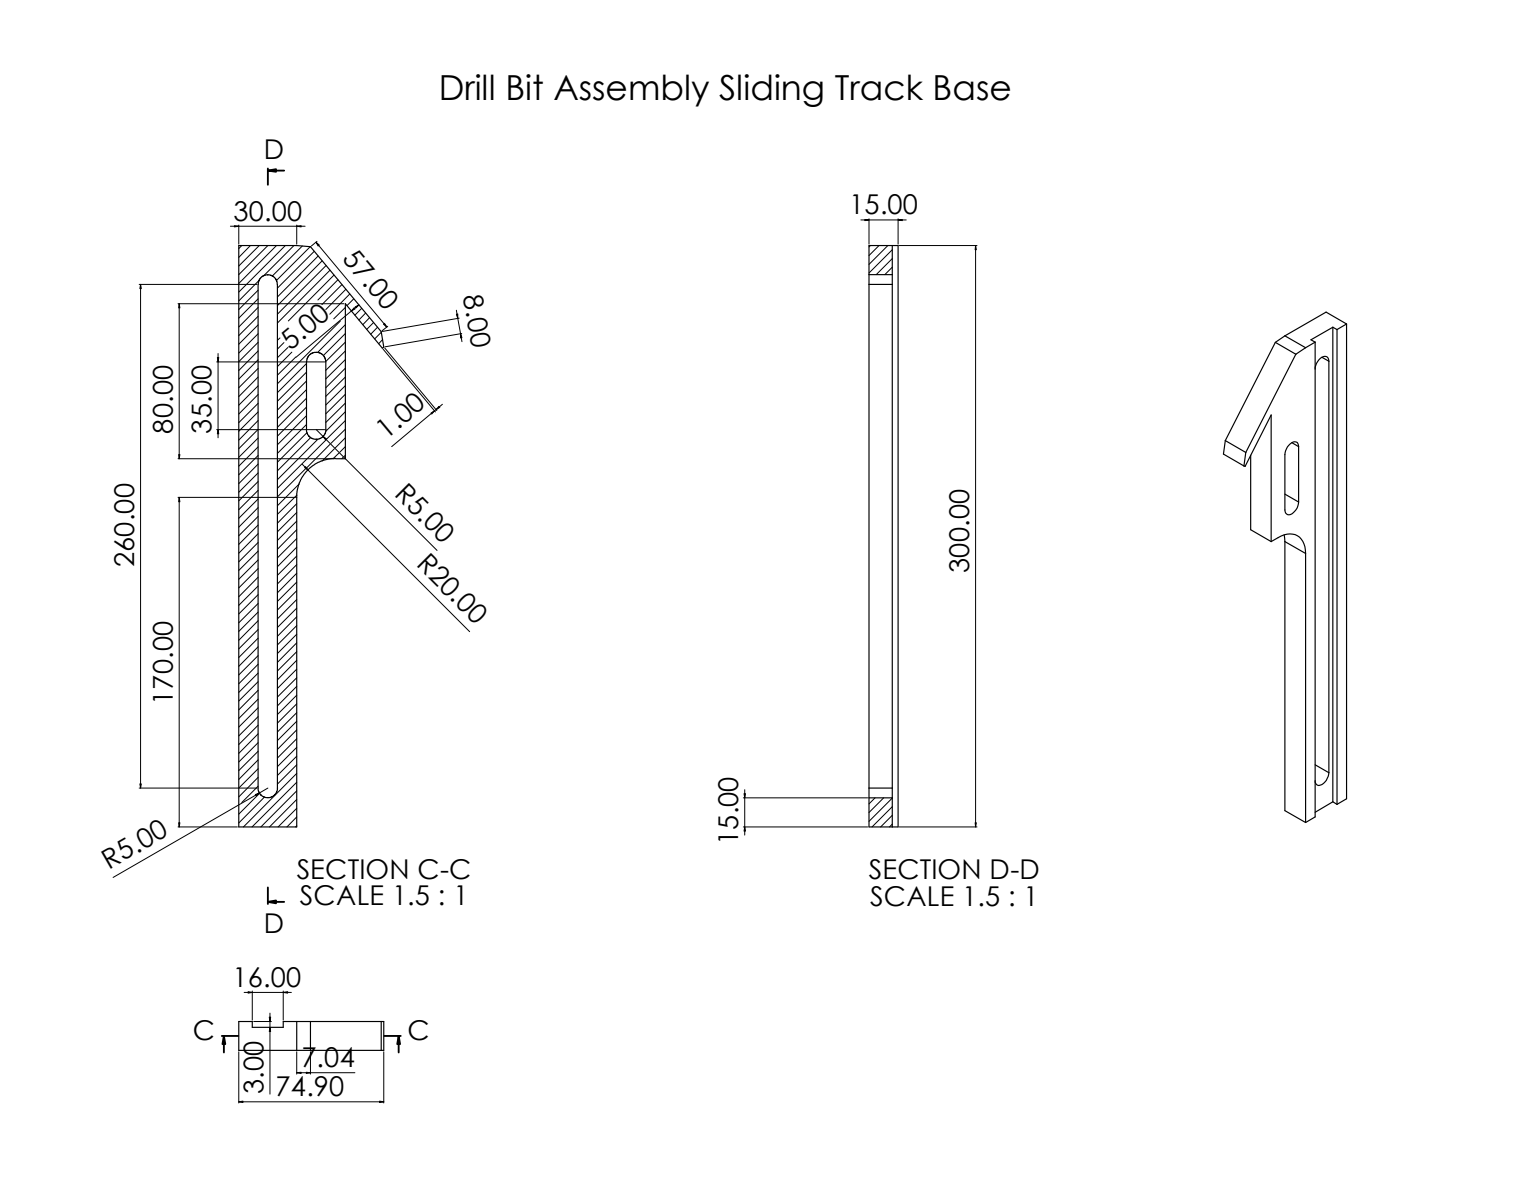
ISO-10303-21;
HEADER;
FILE_DESCRIPTION (('STEP AP214'),
    '1' );
FILE_NAME ('Drill Bit Assembly Sliding Track Base.step',
    '2026-10-26T22:46:44',
    ( '' ),
    ( '' ),
    'SwSTEP 2.0',
    'SolidWorks 2025',
    '' );
FILE_SCHEMA (( 'AUTOMOTIVE_DESIGN' ));
ENDSEC;

DATA;
#10=ORIENTED_EDGE ( 'NONE', *, *, #14818, .T. ) ;
#22=VECTOR ( 'NONE', #7023, 1000.000000000000114 ) ;
#42=CYLINDRICAL_SURFACE ( 'NONE', #6692, 5.000000000000002665 ) ;
#84=AXIS2_PLACEMENT_3D ( 'NONE', #10451, #8972, #10240 ) ;
#92=ORIENTED_EDGE ( 'NONE', *, *, #17549, .F. ) ;
#102=ADVANCED_FACE ( 'NONE', ( #18525 ), #10234, .F. ) ;
#113=ORIENTED_EDGE ( 'NONE', *, *, #4613, .F. ) ;
#117=DIRECTION ( 'NONE',  ( -0.5000000000000029976, 0.8660254037844370423, 0.000000000000000000 ) ) ;
#122=VERTEX_POINT ( 'NONE', #2105 ) ;
#123=APPLICATION_CONTEXT ( 'automotive_design' ) ;
#189=DIRECTION ( 'NONE',  ( -0.8660254037844360431, -0.5000000000000044409, 5.976026924694052093E-17 ) ) ;
#198=PLANE ( 'NONE',  #5711 ) ;
#204=DIRECTION ( 'NONE',  ( 0.8660254037844361541, 0.5000000000000043299, -5.976026924694053325E-17 ) ) ;
#209=ORIENTED_EDGE ( 'NONE', *, *, #20399, .T. ) ;
#222=FACE_OUTER_BOUND ( 'NONE', #14547, .T. ) ;
#243=UNCERTAINTY_MEASURE_WITH_UNIT (LENGTH_MEASURE( 1.000000000000000082E-05 ), #16702, 'distance_accuracy_value', 'NONE');
#300=LINE ( 'NONE', #11651, #4810 ) ;
#312=ORIENTED_EDGE ( 'NONE', *, *, #4694, .F. ) ;
#350=ORIENTED_EDGE ( 'NONE', *, *, #10318, .F. ) ;
#352=CARTESIAN_POINT ( 'NONE',  ( 69.50490953756755630, 173.5703347563769796, 16.00000000000001066 ) ) ;
#362=VECTOR ( 'NONE', #204, 1000.000000000000114 ) ;
#443=ADVANCED_FACE ( 'NONE', ( #4623 ), #13103, .F. ) ;
#466=FACE_OUTER_BOUND ( 'NONE', #2081, .T. ) ;
#469=CARTESIAN_POINT ( 'NONE',  ( 89.99529059433416478, 168.0799536996104848, 21.00000000000000711 ) ) ;
#494=ORIENTED_EDGE ( 'NONE', *, *, #20248, .T. ) ;
#495=FACE_OUTER_BOUND ( 'NONE', #6270, .T. ) ;
#509=ORIENTED_EDGE ( 'NONE', *, *, #2019, .T. ) ;
#517=FACE_OUTER_BOUND ( 'NONE', #17017, .T. ) ;
#524=ORIENTED_EDGE ( 'NONE', *, *, #10776, .F. ) ;
#540=CARTESIAN_POINT ( 'NONE',  ( 52.00490953756739287, 203.8812238888322383, 16.00000000000001066 ) ) ;
#544=DIRECTION ( 'NONE',  ( -1.153604387573317816E-16, 8.028960261725416899E-17, -1.000000000000000000 ) ) ;
#572=LINE ( 'NONE', #11705, #22 ) ;
#596=LINE ( 'NONE', #6053, #2836 ) ;
#604=LINE ( 'NONE', #7163, #17252 ) ;
#614=EDGE_LOOP ( 'NONE', ( #1540, #2040, #6697, #17636 ) ) ;
#640=DIRECTION ( 'NONE',  ( -0.8660254037844361541, -0.5000000000000043299, 0.000000000000000000 ) ) ;
#669=LINE ( 'NONE', #15217, #9538 ) ;
#715=VECTOR ( 'NONE', #14881, 1000.000000000000227 ) ;
#721=DIRECTION ( 'NONE',  ( 0.5000000000000044409, -0.8660254037844360431, -8.673617379884021914E-17 ) ) ;
#734=VERTEX_POINT ( 'NONE', #3213 ) ;
#740=CYLINDRICAL_SURFACE ( 'NONE', #13407, 5.000000000000005329 ) ;
#813=LINE ( 'NONE', #2095, #20345 ) ;
#814=EDGE_CURVE ( 'NONE', #5086, #6648, #7657, .T. ) ;
#817=CARTESIAN_POINT ( 'NONE',  ( 162.0049095375683237, 13.35563505625637859, -19.00000000000000355 ) ) ;
#843=EDGE_CURVE ( 'NONE', #19778, #2748, #14999, .T. ) ;
#873=EDGE_CURVE ( 'NONE', #9960, #7294, #7008, .T. ) ;
#877=AXIS2_PLACEMENT_3D ( 'NONE', #18226, #14549, #1913 ) ;
#909=CARTESIAN_POINT ( 'NONE',  ( 69.50490953756755630, 173.5703347563769796, 6.000000000000010658 ) ) ;
#943=CARTESIAN_POINT ( 'NONE',  ( 57.20986367771971004, 224.8659788670223634, 44.53282986889897899 ) ) ;
#953=ORIENTED_EDGE ( 'NONE', *, *, #3595, .F. ) ;
#988=DIRECTION ( 'NONE',  ( 0.3200921998322429629, -0.5544159532159284032, -0.7682212795973754060 ) ) ;
#1012=ADVANCED_FACE ( 'NONE', ( #2576 ), #12330, .F. ) ;
#1089=( NAMED_UNIT ( * ) PLANE_ANGLE_UNIT ( ) SI_UNIT ( $, .RADIAN. ) );
#1131=LINE ( 'NONE', #10862, #20660 ) ;
#1148=EDGE_CURVE ( 'NONE', #3117, #9960, #12846, .T. ) ;
#1195=DIRECTION ( 'NONE',  ( 0.8660254037844361541, 0.5000000000000043299, -5.976026924694053325E-17 ) ) ;
#1208=VERTEX_POINT ( 'NONE', #4575 ) ;
#1213=DIRECTION ( 'NONE',  ( -0.3841106397986904786, 0.6652991438591134843, -0.6401843996644803747 ) ) ;
#1218=VECTOR ( 'NONE', #4888, 999.9999999999998863 ) ;
#1274=DIRECTION ( 'NONE',  ( 0.000000000000000000, 0.000000000000000000, 1.000000000000000000 ) ) ;
#1325=PRODUCT_DEFINITION_FORMATION_WITH_SPECIFIED_SOURCE ( 'ANY', '', #20237, .NOT_KNOWN. ) ;
#1451=DIRECTION ( 'NONE',  ( -0.5000000000000043299, 0.8660254037844361541, 1.272130549049658454E-16 ) ) ;
#1474=EDGE_CURVE ( 'NONE', #10313, #10227, #2340, .T. ) ;
#1496=ADVANCED_FACE ( 'NONE', ( #13106 ), #11502, .F. ) ;
#1497=DIRECTION ( 'NONE',  ( -0.5000000000000029976, 0.8660254037844370423, 0.000000000000000000 ) ) ;
#1519=CARTESIAN_POINT ( 'NONE',  ( 182.3972143829816446, 2.035126980567696364, -22.00000000000003908 ) ) ;
#1520=CARTESIAN_POINT ( 'NONE',  ( 44.99529059433372424, 246.0222400402097946, -8.999999999999973355 ) ) ;
#1527=ORIENTED_EDGE ( 'NONE', *, *, #14882, .F. ) ;
#1540=ORIENTED_EDGE ( 'NONE', *, *, #15388, .T. ) ;
#1554=ORIENTED_EDGE ( 'NONE', *, *, #5736, .T. ) ;
#1582=EDGE_CURVE ( 'NONE', #4169, #5897, #12618, .T. ) ;
#1650=DIRECTION ( 'NONE',  ( -0.5000000000000029976, 0.8660254037844370423, 0.000000000000000000 ) ) ;
#1712=LINE ( 'NONE', #8374, #13909 ) ;
#1732=EDGE_CURVE ( 'NONE', #16063, #3717, #2384, .T. ) ;
#1744=VERTEX_POINT ( 'NONE', #5228 ) ;
#1750=VECTOR ( 'NONE', #9141, 1000.000000000000114 ) ;
#1757=CARTESIAN_POINT ( 'NONE',  ( 34.99529059433364608, 263.3427481158985302, -28.99999999999997513 ) ) ;
#1792=ORIENTED_EDGE ( 'NONE', *, *, #7559, .F. ) ;
#1808=CARTESIAN_POINT ( 'NONE',  ( 32.39721438298033007, 261.8427481158985302, -22.00000000000000355 ) ) ;
#1848=LINE ( 'NONE', #469, #12796 ) ;
#1871=DIRECTION ( 'NONE',  ( 0.000000000000000000, 0.000000000000000000, -1.000000000000000000 ) ) ;
#1882=VERTEX_POINT ( 'NONE', #18714 ) ;
#1912=AXIS2_PLACEMENT_3D ( 'NONE', #13249, #19798, #11757 ) ;
#1913=DIRECTION ( 'NONE',  ( 0.000000000000000000, -0.8108848540793835991, 0.5852057359806522863 ) ) ;
#1938=EDGE_LOOP ( 'NONE', ( #14408, #7446, #12643, #9895 ) ) ;
#1960=CARTESIAN_POINT ( 'NONE',  ( 57.20986367771984504, 224.8659788670219939, 44.53282986889903583 ) ) ;
#2019=EDGE_CURVE ( 'NONE', #19831, #13880, #17857, .T. ) ;
#2028=ORIENTED_EDGE ( 'NONE', *, *, #7150, .F. ) ;
#2040=ORIENTED_EDGE ( 'NONE', *, *, #1474, .T. ) ;
#2043=ORIENTED_EDGE ( 'NONE', *, *, #1582, .T. ) ;
#2081=EDGE_LOOP ( 'NONE', ( #19123, #6063, #19574, #13979 ) ) ;
#2095=CARTESIAN_POINT ( 'NONE',  ( 184.9952905943349606, 3.535126980567727450, -29.00000000000001066 ) ) ;
#2105=CARTESIAN_POINT ( 'NONE',  ( 48.16104799571871098, 210.5389873765740560, 45.89527237623691747 ) ) ;
#2141=CARTESIAN_POINT ( 'NONE',  ( 32.39721438298033007, 261.8427481158985302, -22.00000000000000355 ) ) ;
#2149=ORIENTED_EDGE ( 'NONE', *, *, #10776, .T. ) ;
#2205=CARTESIAN_POINT ( 'NONE',  ( 99.99529059433426426, 150.7594456239217777, 1.000000000000008438 ) ) ;
#2217=ORIENTED_EDGE ( 'NONE', *, *, #7593, .T. ) ;
#2260=EDGE_CURVE ( 'NONE', #15541, #9504, #13815, .T. ) ;
#2292=EDGE_CURVE ( 'NONE', #9960, #734, #10615, .T. ) ;
#2301=FACE_OUTER_BOUND ( 'NONE', #14390, .T. ) ;
#2312=ORIENTED_EDGE ( 'NONE', *, *, #2928, .T. ) ;
#2340=LINE ( 'NONE', #9202, #6212 ) ;
#2358=ORIENTED_EDGE ( 'NONE', *, *, #1732, .F. ) ;
#2380=DIRECTION ( 'NONE',  ( -0.8660254037844360431, -0.5000000000000044409, 5.976026924694052093E-17 ) ) ;
#2384=LINE ( 'NONE', #15235, #4553 ) ;
#2386=ADVANCED_FACE ( 'NONE', ( #18579 ), #12960, .F. ) ;
#2414=EDGE_CURVE ( 'NONE', #16240, #8157, #16622, .T. ) ;
#2430=CARTESIAN_POINT ( 'NONE',  ( 172.3972143829816162, 19.35563505625646030, -19.00000000000000355 ) ) ;
#2432=ORIENTED_EDGE ( 'NONE', *, *, #4613, .T. ) ;
#2442=VECTOR ( 'NONE', #7671, 1000.000000000000227 ) ;
#2489=ORIENTED_EDGE ( 'NONE', *, *, #3198, .T. ) ;
#2527=PLANE ( 'NONE',  #84 ) ;
#2547=ORIENTED_EDGE ( 'NONE', *, *, #20248, .F. ) ;
#2558=EDGE_CURVE ( 'NONE', #10285, #1208, #19571, .T. ) ;
#2576=FACE_OUTER_BOUND ( 'NONE', #5270, .T. ) ;
#2610=CARTESIAN_POINT ( 'NONE',  ( 87.00490953756771262, 143.2594456239216925, 1.000000000000009326 ) ) ;
#2620=ORIENTED_EDGE ( 'NONE', *, *, #11484, .T. ) ;
#2622=ORIENTED_EDGE ( 'NONE', *, *, #11749, .T. ) ;
#2631=ORIENTED_EDGE ( 'NONE', *, *, #15255, .T. ) ;
#2670=EDGE_LOOP ( 'NONE', ( #8116, #14442, #7233, #8193 ) ) ;
#2748=VERTEX_POINT ( 'NONE', #11956 ) ;
#2768=ORIENTED_EDGE ( 'NONE', *, *, #7687, .T. ) ;
#2775=VECTOR ( 'NONE', #1213, 1000.000000000000114 ) ;
#2780=VECTOR ( 'NONE', #15502, 1000.000000000000227 ) ;
#2836=VECTOR ( 'NONE', #7046, 1000.000000000000227 ) ;
#2837=EDGE_CURVE ( 'NONE', #3359, #10810, #9269, .T. ) ;
#2838=ORIENTED_EDGE ( 'NONE', *, *, #2843, .F. ) ;
#2843=EDGE_CURVE ( 'NONE', #3717, #5485, #15465, .T. ) ;
#2851=APPLICATION_CONTEXT ( 'automotive_design' ) ;
#2854=ORIENTED_EDGE ( 'NONE', *, *, #843, .T. ) ;
#2906=CARTESIAN_POINT ( 'NONE',  ( 22.32500173739930460, 255.2883321626825932, 8.042028396309257587 ) ) ;
#2918=EDGE_LOOP ( 'NONE', ( #509, #20075, #113, #10552 ) ) ;
#2928=EDGE_CURVE ( 'NONE', #2748, #10227, #18337, .T. ) ;
#2955=AXIS2_PLACEMENT_3D ( 'NONE', #19299, #7847, #1497 ) ;
#3005=LINE ( 'NONE', #1519, #7771 ) ;
#3034=LINE ( 'NONE', #15679, #13135 ) ;
#3039=DIRECTION ( 'NONE',  ( 0.5000000000000044409, -0.8660254037844360431, 0.000000000000000000 ) ) ;
#3102=VECTOR ( 'NONE', #7583, 999.9999999999998863 ) ;
#3113=FACE_OUTER_BOUND ( 'NONE', #19423, .T. ) ;
#3117=VERTEX_POINT ( 'NONE', #18277 ) ;
#3186=EDGE_CURVE ( 'NONE', #17982, #10285, #13517, .T. ) ;
#3196=DIRECTION ( 'NONE',  ( -0.8660254037844361541, -0.5000000000000045519, 5.976026924694053325E-17 ) ) ;
#3198=EDGE_CURVE ( 'NONE', #3359, #9504, #10629, .T. ) ;
#3205=CARTESIAN_POINT ( 'NONE',  ( 184.9952905943349606, 3.535126980567709687, -22.00000000000003908 ) ) ;
#3213=CARTESIAN_POINT ( 'NONE',  ( 22.00490953756710510, 255.8427481158984733, -28.99999999999997513 ) ) ;
#3218=ORIENTED_EDGE ( 'NONE', *, *, #843, .F. ) ;
#3232=DIRECTION ( 'NONE',  ( 0.8660254037844360431, 0.5000000000000044409, -5.976026924694053325E-17 ) ) ;
#3270=EDGE_CURVE ( 'NONE', #11034, #20099, #12561, .T. ) ;
#3286=CARTESIAN_POINT ( 'NONE',  ( 52.00490953756739287, 203.8812238888322383, 6.000000000000010658 ) ) ;
#3359=VERTEX_POINT ( 'NONE', #2906 ) ;
#3365=ORIENTED_EDGE ( 'NONE', *, *, #13197, .F. ) ;
#3370=CARTESIAN_POINT ( 'NONE',  ( 44.99529059433372424, 246.0222400402097946, -18.99999999999997513 ) ) ;
#3381=FACE_OUTER_BOUND ( 'NONE', #5314, .T. ) ;
#3390=CARTESIAN_POINT ( 'NONE',  ( 182.3972143829816446, 2.035126980567696364, -6.000000000000009770 ) ) ;
#3405=AXIS2_PLACEMENT_3D ( 'NONE', #14558, #17827, #15934 ) ;
#3412=ORIENTED_EDGE ( 'NONE', *, *, #17197, .F. ) ;
#3415=ORIENTED_EDGE ( 'NONE', *, *, #11618, .F. ) ;
#3417=VECTOR ( 'NONE', #14485, 1000.000000000000227 ) ;
#3440=CARTESIAN_POINT ( 'NONE',  ( 32.00490953756718682, 238.5222400402097094, -13.99999999999997335 ) ) ;
#3441=VECTOR ( 'NONE', #8435, 1000.000000000000114 ) ;
#3470=CARTESIAN_POINT ( 'NONE',  ( 32.00490953756718682, 238.5222400402097094, -18.99999999999997513 ) ) ;
#3473=DIRECTION ( 'NONE',  ( 0.5000000000000044409, -0.8660254037844360431, -8.673617379884021914E-17 ) ) ;
#3494=EDGE_CURVE ( 'NONE', #19831, #15541, #10642, .T. ) ;
#3511=ORIENTED_EDGE ( 'NONE', *, *, #17990, .T. ) ;
#3535=DIRECTION ( 'NONE',  ( 0.5000000000000046629, -0.8660254037844360431, 0.000000000000000000 ) ) ;
#3546=DIRECTION ( 'NONE',  ( -0.3200921998322431850, 0.5544159532159285142, 0.7682212795973754060 ) ) ;
#3559=AXIS2_PLACEMENT_3D ( 'NONE', #18463, #13907, #10606 ) ;
#3595=EDGE_CURVE ( 'NONE', #6648, #16240, #11289, .T. ) ;
#3609=CARTESIAN_POINT ( 'NONE',  ( 32.39721438298033007, 261.8427481158985302, -5.999999999999973355 ) ) ;
#3613=CARTESIAN_POINT ( 'NONE',  ( 46.88067919638974956, 212.7566511894377754, 48.96815749462641065 ) ) ;
#3644=( GEOMETRIC_REPRESENTATION_CONTEXT ( 3 ) GLOBAL_UNCERTAINTY_ASSIGNED_CONTEXT ( ( #16361 ) ) GLOBAL_UNIT_ASSIGNED_CONTEXT ( ( #12219, #1089, #15522 ) ) REPRESENTATION_CONTEXT ( 'NONE', 'WORKASPACE' ) );
#3645=( NAMED_UNIT ( * ) SI_UNIT ( $, .STERADIAN. ) SOLID_ANGLE_UNIT ( ) );
#3648=VECTOR ( 'NONE', #4240, 1000.000000000000227 ) ;
#3663=LINE ( 'NONE', #11635, #7812 ) ;
#3681=CARTESIAN_POINT ( 'NONE',  ( 32.39721438298033007, 261.8427481158985302, -5.999999999999973355 ) ) ;
#3705=VECTOR ( 'NONE', #20609, 1000.000000000000000 ) ;
#3717=VERTEX_POINT ( 'NONE', #18167 ) ;
#3723=DIRECTION ( 'NONE',  ( 0.5000000000000058842, -0.8660254037844352659, 0.000000000000000000 ) ) ;
#3735=ORIENTED_EDGE ( 'NONE', *, *, #4294, .F. ) ;
#3757=VERTEX_POINT ( 'NONE', #5535 ) ;
#3758=AXIS2_PLACEMENT_3D ( 'NONE', #9685, #6391, #3535 ) ;
#3776=DIRECTION ( 'NONE',  ( -0.000000000000000000, 4.625929269271485914E-16, -1.000000000000000000 ) ) ;
#3810=VERTEX_POINT ( 'NONE', #13932 ) ;
#3831=ORIENTED_EDGE ( 'NONE', *, *, #4082, .F. ) ;
#3868=CARTESIAN_POINT ( 'NONE',  ( -104.9618400369722622, 181.7992397999509819, 8.042028396309241600 ) ) ;
#3914=AXIS2_PLACEMENT_3D ( 'NONE', #15936, #4983, #4679 ) ;
#3939=AXIS2_PLACEMENT_3D ( 'NONE', #13181, #18468, #3723 ) ;
#4015=DIRECTION ( 'NONE',  ( 0.5000000000000041078, -0.8660254037844363761, 0.000000000000000000 ) ) ;
#4052=CARTESIAN_POINT ( 'NONE',  ( 82.49529059433407951, 181.0703347563770365, 16.00000000000001066 ) ) ;
#4065=CARTESIAN_POINT ( 'NONE',  ( 35.31538279416584913, 262.7883321626826501, 8.042028396309257587 ) ) ;
#4082=EDGE_CURVE ( 'NONE', #3117, #5485, #13375, .T. ) ;
#4118=ORIENTED_EDGE ( 'NONE', *, *, #3198, .F. ) ;
#4169=VERTEX_POINT ( 'NONE', #18359 ) ;
#4188=LINE ( 'NONE', #20716, #2442 ) ;
#4191=ORIENTED_EDGE ( 'NONE', *, *, #6008, .F. ) ;
#4205=CARTESIAN_POINT ( 'NONE',  ( 184.9952905943349606, 3.535126980567713240, 0.9999999999999876765 ) ) ;
#4220=LINE ( 'NONE', #5477, #17086 ) ;
#4239=CARTESIAN_POINT ( 'NONE',  ( 32.00490953756718682, 238.5222400402097094, -8.999999999999971578 ) ) ;
#4240=DIRECTION ( 'NONE',  ( -0.8660254037844360431, -0.5000000000000044409, 5.976026924694052093E-17 ) ) ;
#4294=EDGE_CURVE ( 'NONE', #3810, #16846, #9187, .T. ) ;
#4326=ORIENTED_EDGE ( 'NONE', *, *, #13282, .T. ) ;
#4364=CARTESIAN_POINT ( 'NONE',  ( 34.99529059433364608, 263.3427481158985302, -28.99999999999997513 ) ) ;
#4378=ORIENTED_EDGE ( 'NONE', *, *, #16152, .T. ) ;
#4400=CARTESIAN_POINT ( 'NONE',  ( 174.9952905943348469, 20.85563505625644609, -9.000000000000007105 ) ) ;
#4411=CARTESIAN_POINT ( 'NONE',  ( 20.40444853840588380, 258.6148278819781012, 4.841106397986906451 ) ) ;
#4439=DIRECTION ( 'NONE',  ( -5.175391130484829193E-17, -2.988013462347053780E-17, -1.000000000000000000 ) ) ;
#4475=ORIENTED_EDGE ( 'NONE', *, *, #4694, .T. ) ;
#4549=AXIS2_PLACEMENT_3D ( 'NONE', #12070, #20323, #10454 ) ;
#4553=VECTOR ( 'NONE', #16703, 1000.000000000000227 ) ;
#4575=CARTESIAN_POINT ( 'NONE',  ( 37.00490953756721524, 229.8619860023653985, 26.00000000000001776 ) ) ;
#4592=EDGE_CURVE ( 'NONE', #8802, #3117, #813, .T. ) ;
#4605=LINE ( 'NONE', #2610, #5814 ) ;
#4613=EDGE_CURVE ( 'NONE', #13544, #16413, #604, .T. ) ;
#4623=FACE_OUTER_BOUND ( 'NONE', #13097, .T. ) ;
#4629=FACE_OUTER_BOUND ( 'NONE', #14208, .T. ) ;
#4633=LINE ( 'NONE', #19160, #19626 ) ;
#4672=DIRECTION ( 'NONE',  ( -0.5000000000000043299, 0.8660254037844361541, 1.272130549049658700E-16 ) ) ;
#4679=DIRECTION ( 'NONE',  ( 0.5000000000000046629, -0.8660254037844360431, 0.000000000000000000 ) ) ;
#4693=ORIENTED_EDGE ( 'NONE', *, *, #10164, .T. ) ;
#4694=EDGE_CURVE ( 'NONE', #16413, #17073, #3005, .T. ) ;
#4720=DIRECTION ( 'NONE',  ( -0.5000000000000041078, 0.8660254037844363761, 0.000000000000000000 ) ) ;
#4770=AXIS2_PLACEMENT_3D ( 'NONE', #3868, #5657, #16709 ) ;
#4804=FACE_OUTER_BOUND ( 'NONE', #9235, .T. ) ;
#4810=VECTOR ( 'NONE', #18113, 1000.000000000000114 ) ;
#4818=ORIENTED_EDGE ( 'NONE', *, *, #16276, .F. ) ;
#4828=FACE_OUTER_BOUND ( 'NONE', #14732, .T. ) ;
#4862=DIRECTION ( 'NONE',  ( 0.5000000000000042188, -0.8660254037844361541, -1.067522139062650425E-16 ) ) ;
#4888=DIRECTION ( 'NONE',  ( 0.3841106397986906451, -0.6652991438591134843, 0.6401843996644803747 ) ) ;
#4948=DIRECTION ( 'NONE',  ( -0.5000000000000029976, 0.8660254037844370423, 0.000000000000000000 ) ) ;
#4983=DIRECTION ( 'NONE',  ( -0.8660254037844361541, -0.5000000000000045519, 5.976026924694053325E-17 ) ) ;
#5016=ORIENTED_EDGE ( 'NONE', *, *, #14063, .T. ) ;
#5082=CARTESIAN_POINT ( 'NONE',  ( 22.00490953756709800, 255.8427481158984733, 1.000000000000028644 ) ) ;
#5086=VERTEX_POINT ( 'NONE', #17294 ) ;
#5161=DIRECTION ( 'NONE',  ( 1.000000000000000000, 0.000000000000000000, -1.051300182579813185E-16 ) ) ;
#5198=ORIENTED_EDGE ( 'NONE', *, *, #9866, .T. ) ;
#5220=ORIENTED_EDGE ( 'NONE', *, *, #17144, .T. ) ;
#5221=DIRECTION ( 'NONE',  ( 0.8660254037844370423, 0.5000000000000027756, 1.765692291717890446E-15 ) ) ;
#5228=CARTESIAN_POINT ( 'NONE',  ( 77.00490953756764156, 160.5799536996104280, 26.00000000000001066 ) ) ;
#5229=ORIENTED_EDGE ( 'NONE', *, *, #1474, .F. ) ;
#5234=VERTEX_POINT ( 'NONE', #13676 ) ;
#5270=EDGE_LOOP ( 'NONE', ( #5198, #20606, #18436, #10211 ) ) ;
#5314=EDGE_LOOP ( 'NONE', ( #14238, #12408, #12374, #6867 ) ) ;
#5327=STYLED_ITEM('',(#20967),#17741);
#5428=CARTESIAN_POINT ( 'NONE',  ( 64.99529059433392320, 211.3812238888322952, 6.000000000000009770 ) ) ;
#5446=CARTESIAN_POINT ( 'NONE',  ( 61.15142905248526262, 218.0389873765740845, 45.89527237623694589 ) ) ;
#5454=DIRECTION ( 'NONE',  ( 0.5000000000000043299, -0.8660254037844361541, -1.214306433183764966E-16 ) ) ;
#5456=VECTOR ( 'NONE', #15711, 1000.000000000000000 ) ;
#5470=DIRECTION ( 'NONE',  ( -0.8660254037844361541, -0.5000000000000045519, 5.976026924694053325E-17 ) ) ;
#5477=CARTESIAN_POINT ( 'NONE',  ( 32.39721438298033007, 261.8427481158985302, -22.00000000000000355 ) ) ;
#5485=VERTEX_POINT ( 'NONE', #7817 ) ;
#5487=CARTESIAN_POINT ( 'NONE',  ( 34.99529059433364608, 263.3427481158985302, 1.000000000000028644 ) ) ;
#5503=ADVANCED_FACE ( 'NONE', ( #7612 ), #20539, .T. ) ;
#5535=CARTESIAN_POINT ( 'NONE',  ( 87.00490953756771262, 143.2594456239216925, 1.000000000000007772 ) ) ;
#5546=AXIS2_PLACEMENT_3D ( 'NONE', #17980, #3546, #10913 ) ;
#5551=EDGE_LOOP ( 'NONE', ( #2149, #11995, #3511, #13734, #2622 ) ) ;
#5580=PLANE ( 'NONE',  #4549 ) ;
#5611=VECTOR ( 'NONE', #11972, 1000.000000000000114 ) ;
#5613=EDGE_CURVE ( 'NONE', #10227, #20099, #17306, .T. ) ;
#5616=DIRECTION ( 'NONE',  ( -0.000000000000000000, 4.625929269271485914E-16, -1.000000000000000000 ) ) ;
#5657=DIRECTION ( 'NONE',  ( -0.4979466032338565329, 0.8624688162573705963, 0.09053574604251182767 ) ) ;
#5673=DIRECTION ( 'NONE',  ( -0.000000000000000000, 4.625929269271485914E-16, -1.000000000000000000 ) ) ;
#5678=CARTESIAN_POINT ( 'NONE',  ( 82.49529059433407951, 181.0703347563770365, 6.000000000000009770 ) ) ;
#5700=LINE ( 'NONE', #20448, #3648 ) ;
#5701=DIRECTION ( 'NONE',  ( -0.8660254037844360431, -0.5000000000000044409, 5.976026924694052093E-17 ) ) ;
#5704=CARTESIAN_POINT ( 'NONE',  ( 69.50490953756755630, 173.5703347563769796, 6.000000000000010658 ) ) ;
#5711=AXIS2_PLACEMENT_3D ( 'NONE', #11649, #6640, #14949 ) ;
#5736=EDGE_CURVE ( 'NONE', #13841, #3757, #16072, .T. ) ;
#5750=LINE ( 'NONE', #15550, #16856 ) ;
#5794=DIRECTION ( 'NONE',  ( -0.5000000000000041078, 0.8660254037844363761, 0.000000000000000000 ) ) ;
#5797=ORIENTED_EDGE ( 'NONE', *, *, #11749, .F. ) ;
#5814=VECTOR ( 'NONE', #7564, 1000.000000000000227 ) ;
#5883=CARTESIAN_POINT ( 'NONE',  ( 32.39721438298033007, 261.8427481158985302, -22.00000000000000355 ) ) ;
#5897=VERTEX_POINT ( 'NONE', #4052 ) ;
#5900=CARTESIAN_POINT ( 'NONE',  ( 44.99529059433372424, 246.0222400402097946, -8.999999999999973355 ) ) ;
#5901=ORIENTED_EDGE ( 'NONE', *, *, #11594, .F. ) ;
#5912=EDGE_CURVE ( 'NONE', #11034, #11090, #669, .T. ) ;
#5933=AXIS2_PLACEMENT_3D ( 'NONE', #11262, #3196, #6253 ) ;
#5957=VECTOR ( 'NONE', #17242, 1000.000000000000114 ) ;
#5959=CARTESIAN_POINT ( 'NONE',  ( 23.43933576707516053, 253.3582490066810919, 32.55737704917950737 ) ) ;
#5991=CARTESIAN_POINT ( 'NONE',  ( 57.20986367771982373, 224.8659788670219655, 44.53282986889902162 ) ) ;
#6008=EDGE_CURVE ( 'NONE', #14393, #17982, #7231, .T. ) ;
#6019=DIRECTION ( 'NONE',  ( 0.5000000000000045519, -0.8660254037844360431, -0.000000000000000000 ) ) ;
#6053=CARTESIAN_POINT ( 'NONE',  ( 82.49529059433407951, 181.0703347563770365, 16.00000000000001066 ) ) ;
#6060=DIRECTION ( 'NONE',  ( -1.218100516808353647E-16, 9.146065988991504310E-17, -1.000000000000000000 ) ) ;
#6063=ORIENTED_EDGE ( 'NONE', *, *, #8198, .F. ) ;
#6074=ORIENTED_EDGE ( 'NONE', *, *, #4294, .T. ) ;
#6161=VECTOR ( 'NONE', #1195, 1000.000000000000114 ) ;
#6212=VECTOR ( 'NONE', #5701, 1000.000000000000227 ) ;
#6253=DIRECTION ( 'NONE',  ( 0.5000000000000029976, -0.8660254037844370423, 0.000000000000000000 ) ) ;
#6270=EDGE_LOOP ( 'NONE', ( #8550, #16847, #4118, #350 ) ) ;
#6328=CARTESIAN_POINT ( 'NONE',  ( 32.00490953756718682, 238.5222400402097094, -8.999999999999971578 ) ) ;
#6341=ORIENTED_EDGE ( 'NONE', *, *, #7687, .F. ) ;
#6363=AXIS2_PLACEMENT_3D ( 'NONE', #1520, #6060, #12554 ) ;
#6370=ORIENTED_EDGE ( 'NONE', *, *, #18466, .F. ) ;
#6391=DIRECTION ( 'NONE',  ( -0.8660254037844360431, -0.5000000000000044409, 5.976026924694053325E-17 ) ) ;
#6439=CARTESIAN_POINT ( 'NONE',  ( 99.99529059433426426, 150.7594456239217777, 1.000000000000006883 ) ) ;
#6447=VECTOR ( 'NONE', #189, 1000.000000000000227 ) ;
#6481=CARTESIAN_POINT ( 'NONE',  ( 174.9952905943348469, 20.85563505625644609, -14.00000000000000533 ) ) ;
#6528=CARTESIAN_POINT ( 'NONE',  ( 37.00490953756721524, 229.8619860023653985, 26.00000000000001776 ) ) ;
#6539=VECTOR ( 'NONE', #4672, 1000.000000000000227 ) ;
#6554=VECTOR ( 'NONE', #6019, 1000.000000000000227 ) ;
#6572=CARTESIAN_POINT ( 'NONE',  ( 184.9952905943349606, 3.535126980567727450, -29.00000000000001066 ) ) ;
#6640=DIRECTION ( 'NONE',  ( -0.8660254037844361541, -0.5000000000000045519, 5.976026924694054558E-17 ) ) ;
#6648=VERTEX_POINT ( 'NONE', #18191 ) ;
#6665=LINE ( 'NONE', #16143, #15111 ) ;
#6692=AXIS2_PLACEMENT_3D ( 'NONE', #6481, #12982, #17855 ) ;
#6697=ORIENTED_EDGE ( 'NONE', *, *, #2928, .F. ) ;
#6731=ORIENTED_EDGE ( 'NONE', *, *, #7773, .T. ) ;
#6734=CARTESIAN_POINT ( 'NONE',  ( 69.50490953756755630, 173.5703347563769796, 11.00000000000001243 ) ) ;
#6745=CARTESIAN_POINT ( 'NONE',  ( 42.39721438298049350, 244.5222400402098231, -18.99999999999997513 ) ) ;
#6756=VECTOR ( 'NONE', #12549, 1000.000000000000000 ) ;
#6819=ADVANCED_FACE ( 'NONE', ( #495 ), #20194, .T. ) ;
#6827=VECTOR ( 'NONE', #13191, 1000.000000000000114 ) ;
#6832=DIRECTION ( 'NONE',  ( -9.512199820426880209E-17, 4.523559531338709945E-17, -1.000000000000000000 ) ) ;
#6867=ORIENTED_EDGE ( 'NONE', *, *, #10318, .T. ) ;
#6910=CARTESIAN_POINT ( 'NONE',  ( 99.99529059433426426, 150.7594456239217777, 21.00000000000000711 ) ) ;
#6962=CYLINDRICAL_SURFACE ( 'NONE', #11146, 5.000000000000001776 ) ;
#6985=PLANE ( 'NONE',  #9436 ) ;
#7008=LINE ( 'NONE', #14890, #9679 ) ;
#7018=AXIS2_PLACEMENT_3D ( 'NONE', #9893, #6832, #19547 ) ;
#7023=DIRECTION ( 'NONE',  ( 0.04526787302125637180, -0.07840625602339144906, 0.9958932064677044060 ) ) ;
#7046=DIRECTION ( 'NONE',  ( -0.8660254037844360431, -0.5000000000000044409, 5.976026924694052093E-17 ) ) ;
#7066=DIRECTION ( 'NONE',  ( -1.000000000000000000, 0.000000000000000000, 1.129794457510891260E-16 ) ) ;
#7067=CARTESIAN_POINT ( 'NONE',  ( 177.4952905943348753, 16.52550803733426577, -14.00000000000000533 ) ) ;
#7081=ORIENTED_EDGE ( 'NONE', *, *, #2558, .T. ) ;
#7095=DIRECTION ( 'NONE',  ( -0.5000000000000041078, 0.8660254037844363761, 0.000000000000000000 ) ) ;
#7117=DIRECTION ( 'NONE',  ( -0.8660254037844361541, -0.5000000000000045519, 5.976026924694053325E-17 ) ) ;
#7150=EDGE_CURVE ( 'NONE', #14393, #122, #1712, .T. ) ;
#7160=ORIENTED_EDGE ( 'NONE', *, *, #9514, .T. ) ;
#7163=CARTESIAN_POINT ( 'NONE',  ( 32.39721438298033007, 261.8427481158985302, -5.999999999999973355 ) ) ;
#7172=PRODUCT_DEFINITION ( 'UNKNOWN', '', #1325, #12355 ) ;
#7193=FACE_OUTER_BOUND ( 'NONE', #11584, .T. ) ;
#7212=FACE_OUTER_BOUND ( 'NONE', #8758, .T. ) ;
#7217=ORIENTED_EDGE ( 'NONE', *, *, #14063, .F. ) ;
#7219=LINE ( 'NONE', #20152, #10683 ) ;
#7231=LINE ( 'NONE', #18584, #12283 ) ;
#7233=ORIENTED_EDGE ( 'NONE', *, *, #5912, .T. ) ;
#7234=AXIS2_PLACEMENT_3D ( 'NONE', #4364, #18894, #20366 ) ;
#7294=VERTEX_POINT ( 'NONE', #7520 ) ;
#7386=DIRECTION ( 'NONE',  ( 0.4926956718456823592, -0.8533739363059945626, 0.1703053134172390071 ) ) ;
#7402=LINE ( 'NONE', #5704, #2780 ) ;
#7440=CARTESIAN_POINT ( 'NONE',  ( 61.47152125231750830, 217.4845714233581475, 45.12705109663956193 ) ) ;
#7446=ORIENTED_EDGE ( 'NONE', *, *, #2558, .F. ) ;
#7493=VECTOR ( 'NONE', #5221, 1000.000000000000000 ) ;
#7510=VECTOR ( 'NONE', #7774, 1000.000000000000227 ) ;
#7520=CARTESIAN_POINT ( 'NONE',  ( 34.99529059433363898, 263.3427481158985302, -22.00000000000000355 ) ) ;
#7540=LINE ( 'NONE', #20159, #16781 ) ;
#7546=ORIENTED_EDGE ( 'NONE', *, *, #18466, .T. ) ;
#7559=EDGE_CURVE ( 'NONE', #13544, #19831, #14750, .T. ) ;
#7564=DIRECTION ( 'NONE',  ( 0.5000000000000043299, -0.8660254037844361541, -1.224510688924805588E-16 ) ) ;
#7583=DIRECTION ( 'NONE',  ( 0.3841106397986906451, -0.6652991438591134843, 0.6401843996644803747 ) ) ;
#7593=EDGE_CURVE ( 'NONE', #11291, #19778, #9148, .T. ) ;
#7612=FACE_OUTER_BOUND ( 'NONE', #12837, .T. ) ;
#7657=CIRCLE ( 'NONE', #3939, 5.000000000000001776 ) ;
#7659=PLANE ( 'NONE',  #6363 ) ;
#7664=CARTESIAN_POINT ( 'NONE',  ( 82.49529059433407951, 181.0703347563770365, 6.000000000000009770 ) ) ;
#7671=DIRECTION ( 'NONE',  ( 0.5000000000000043299, -0.8660254037844361541, -1.224510688924805588E-16 ) ) ;
#7687=EDGE_CURVE ( 'NONE', #16560, #13544, #4220, .T. ) ;
#7699=ADVANCED_FACE ( 'NONE', ( #15274 ), #5580, .T. ) ;
#7737=ORIENTED_EDGE ( 'NONE', *, *, #11594, .T. ) ;
#7771=VECTOR ( 'NONE', #16154, 1000.000000000000000 ) ;
#7773=EDGE_CURVE ( 'NONE', #4169, #19778, #4633, .T. ) ;
#7774=DIRECTION ( 'NONE',  ( -0.8660254037844360431, -0.5000000000000044409, 5.976026924694052093E-17 ) ) ;
#7812=VECTOR ( 'NONE', #10115, 1000.000000000000114 ) ;
#7817=CARTESIAN_POINT ( 'NONE',  ( 172.0049095375684090, -3.964873019432338275, -29.00000000000001066 ) ) ;
#7847=DIRECTION ( 'NONE',  ( 0.8660254037844360431, 0.5000000000000044409, -5.976026924694053325E-17 ) ) ;
#7953=CARTESIAN_POINT ( 'NONE',  ( 184.9952905943349606, 3.535126980567727450, -29.00000000000001066 ) ) ;
#7981=DIRECTION ( 'NONE',  ( 0.5000000000000043299, -0.8660254037844361541, -1.214306433183764966E-16 ) ) ;
#8000=CIRCLE ( 'NONE', #2955, 5.000000000000001776 ) ;
#8038=CARTESIAN_POINT ( 'NONE',  ( 82.49529059433407951, 181.0703347563770365, 11.00000000000001066 ) ) ;
#8071=AXIS2_PLACEMENT_3D ( 'NONE', #9944, #8367, #7095 ) ;
#8073=DIRECTION ( 'NONE',  ( 0.3200921998322429629, -0.5544159532159284032, -0.7682212795973754060 ) ) ;
#8079=DIRECTION ( 'NONE',  ( 0.8660254037844360431, 0.5000000000000044409, -5.976026924694053325E-17 ) ) ;
#8114=VECTOR ( 'NONE', #15828, 1000.000000000000227 ) ;
#8116=ORIENTED_EDGE ( 'NONE', *, *, #9977, .F. ) ;
#8133=CARTESIAN_POINT ( 'NONE',  ( 49.99529059433370293, 237.3619860023655121, 26.00000000000001066 ) ) ;
#8157=VERTEX_POINT ( 'NONE', #12152 ) ;
#8193=ORIENTED_EDGE ( 'NONE', *, *, #17197, .T. ) ;
#8198=EDGE_CURVE ( 'NONE', #8802, #7294, #1131, .T. ) ;
#8200=CARTESIAN_POINT ( 'NONE',  ( 69.50490953756755630, 173.5703347563769796, 11.00000000000001243 ) ) ;
#8279=DIRECTION ( 'NONE',  ( 0.5000000000000045519, -0.8660254037844360431, -0.000000000000000000 ) ) ;
#8330=EDGE_LOOP ( 'NONE', ( #19170, #13459, #312, #14094, #15891, #12655, #14236, #3831 ) ) ;
#8344=FACE_BOUND ( 'NONE', #17345, .T. ) ;
#8352=CIRCLE ( 'NONE', #18170, 5.000000000000005329 ) ;
#8353=ORIENTED_EDGE ( 'NONE', *, *, #5613, .F. ) ;
#8367=DIRECTION ( 'NONE',  ( 0.8660254037844360431, 0.5000000000000044409, -5.976026924694053325E-17 ) ) ;
#8374=CARTESIAN_POINT ( 'NONE',  ( 48.16104799571871098, 210.5389873765740560, 45.89527237623691747 ) ) ;
#8395=MECHANICAL_DESIGN_GEOMETRIC_PRESENTATION_REPRESENTATION('',(#5327),#3644);
#8429=ORIENTED_EDGE ( 'NONE', *, *, #8594, .T. ) ;
#8435=DIRECTION ( 'NONE',  ( -0.5000000000000043299, 0.8660254037844361541, 1.067522139062650548E-16 ) ) ;
#8448=PLANE ( 'NONE',  #11930 ) ;
#8473=AXIS2_PLACEMENT_3D ( 'NONE', #3613, #10671, #10065 ) ;
#8499=ORIENTED_EDGE ( 'NONE', *, *, #3494, .F. ) ;
#8530=SHAPE_REPRESENTATION_RELATIONSHIP ( 'NONE' , 'NONE' ,  #20473, #19205 ) ;
#8550=ORIENTED_EDGE ( 'NONE', *, *, #8594, .F. ) ;
#8551=DIRECTION ( 'NONE',  ( -0.8660254037844360431, -0.5000000000000043299, 0.000000000000000000 ) ) ;
#8557=CARTESIAN_POINT ( 'NONE',  ( 64.99529059433392320, 211.3812238888322952, 6.000000000000009770 ) ) ;
#8594=EDGE_CURVE ( 'NONE', #15541, #11249, #572, .T. ) ;
#8657=CARTESIAN_POINT ( 'NONE',  ( 42.39721438298049350, 244.5222400402098231, -13.99999999999997513 ) ) ;
#8689=DIRECTION ( 'NONE',  ( 0.8660254037844361541, 0.5000000000000043299, -5.976026924694053325E-17 ) ) ;
#8711=EDGE_CURVE ( 'NONE', #5234, #16498, #10834, .T. ) ;
#8758=EDGE_LOOP ( 'NONE', ( #19563, #14565, #13610, #20431 ) ) ;
#8802=VERTEX_POINT ( 'NONE', #3205 ) ;
#8848=VERTEX_POINT ( 'NONE', #2430 ) ;
#8866=ADVANCED_FACE ( 'NONE', ( #18643 ), #13276, .F. ) ;
#8875=FACE_OUTER_BOUND ( 'NONE', #2918, .T. ) ;
#8915=FACE_OUTER_BOUND ( 'NONE', #16105, .T. ) ;
#8972=DIRECTION ( 'NONE',  ( 1.124692329640370702E-16, -7.528188728813031952E-17, 1.000000000000000000 ) ) ;
#8983=ORIENTED_EDGE ( 'NONE', *, *, #2837, .F. ) ;
#8987=DIRECTION ( 'NONE',  ( -0.8660254037844361541, -0.5000000000000045519, 5.976026924694053325E-17 ) ) ;
#8990=AXIS2_PLACEMENT_3D ( 'NONE', #8038, #9738, #117 ) ;
#9033=CARTESIAN_POINT ( 'NONE',  ( 89.99529059433416478, 168.0799536996104848, 26.00000000000001066 ) ) ;
#9036=DIRECTION ( 'NONE',  ( -0.5000000000000043299, 0.8660254037844361541, 1.272130549049658700E-16 ) ) ;
#9141=DIRECTION ( 'NONE',  ( -0.04526787302125637180, 0.07840625602339144906, -0.9958932064677044060 ) ) ;
#9145=EDGE_CURVE ( 'NONE', #122, #10810, #3663, .T. ) ;
#9148=CIRCLE ( 'NONE', #11876, 5.000000000000005329 ) ;
#9187=LINE ( 'NONE', #5900, #11540 ) ;
#9202=CARTESIAN_POINT ( 'NONE',  ( 84.99529059433409373, 176.7402077374548526, 11.00000000000001066 ) ) ;
#9235=EDGE_LOOP ( 'NONE', ( #13280, #16164, #18602, #2547 ) ) ;
#9269=LINE ( 'NONE', #4411, #3102 ) ;
#9315=VECTOR ( 'NONE', #8689, 1000.000000000000114 ) ;
#9333=ADVANCED_FACE ( 'NONE', ( #2301 ), #12054, .F. ) ;
#9341=VECTOR ( 'NONE', #8279, 1000.000000000000227 ) ;
#9436=AXIS2_PLACEMENT_3D ( 'NONE', #11774, #640, #14767 ) ;
#9504=VERTEX_POINT ( 'NONE', #9783 ) ;
#9506=ORIENTED_EDGE ( 'NONE', *, *, #11620, .F. ) ;
#9514=EDGE_CURVE ( 'NONE', #16498, #13841, #18661, .T. ) ;
#9538=VECTOR ( 'NONE', #18480, 1000.000000000000227 ) ;
#9630=EDGE_LOOP ( 'NONE', ( #2620, #13360, #20109, #12526, #494 ) ) ;
#9679=VECTOR ( 'NONE', #13495, 1000.000000000000000 ) ;
#9685=CARTESIAN_POINT ( 'NONE',  ( 99.99529059433426426, 150.7594456239217777, 21.00000000000000711 ) ) ;
#9710=ORIENTED_EDGE ( 'NONE', *, *, #14818, .F. ) ;
#9738=DIRECTION ( 'NONE',  ( 0.8660254037844360431, 0.5000000000000044409, -5.976026924694053325E-17 ) ) ;
#9783=CARTESIAN_POINT ( 'NONE',  ( 22.00490953756709800, 255.8427481158984733, 1.000000000000028644 ) ) ;
#9814=CARTESIAN_POINT ( 'NONE',  ( 49.99529059433375267, 237.3619860023654553, 26.00000000000001776 ) ) ;
#9848=CYLINDRICAL_SURFACE ( 'NONE', #5933, 5.000000000000001776 ) ;
#9866=EDGE_CURVE ( 'NONE', #5485, #734, #10730, .T. ) ;
#9872=AXIS2_PLACEMENT_3D ( 'NONE', #6910, #12016, #18377 ) ;
#9893=CARTESIAN_POINT ( 'NONE',  ( 49.99529059433375267, 237.3619860023654553, 26.00000000000001776 ) ) ;
#9895=ORIENTED_EDGE ( 'NONE', *, *, #19505, .F. ) ;
#9904=CARTESIAN_POINT ( 'NONE',  ( 77.00490953756764156, 160.5799536996104280, 26.00000000000001066 ) ) ;
#9913=ORIENTED_EDGE ( 'NONE', *, *, #17144, .F. ) ;
#9944=CARTESIAN_POINT ( 'NONE',  ( 64.99529059433392320, 211.3812238888322952, 11.00000000000001066 ) ) ;
#9960=VERTEX_POINT ( 'NONE', #20140 ) ;
#9974=DIRECTION ( 'NONE',  ( -0.8660254037844360431, -0.5000000000000044409, 5.976026924694052093E-17 ) ) ;
#9977=EDGE_CURVE ( 'NONE', #20099, #11291, #7402, .T. ) ;
#10065=DIRECTION ( 'NONE',  ( 0.000000000000000000, 0.6933752452815372669, 0.7205766921228913269 ) ) ;
#10115=DIRECTION ( 'NONE',  ( -0.4926956718456823592, 0.8533739363059945626, -0.1703053134172390071 ) ) ;
#10124=CARTESIAN_POINT ( 'NONE',  ( 182.3972143829816446, 2.035126980567696364, -22.00000000000003908 ) ) ;
#10138=EDGE_LOOP ( 'NONE', ( #19239, #2028, #11217, #11110 ) ) ;
#10164=EDGE_CURVE ( 'NONE', #734, #9504, #17176, .T. ) ;
#10178=AXIS2_PLACEMENT_3D ( 'NONE', #6734, #16108, #4948 ) ;
#10190=VECTOR ( 'NONE', #4862, 1000.000000000000114 ) ;
#10198=VECTOR ( 'NONE', #2380, 1000.000000000000227 ) ;
#10211=ORIENTED_EDGE ( 'NONE', *, *, #4082, .T. ) ;
#10227=VERTEX_POINT ( 'NONE', #19387 ) ;
#10234=PLANE ( 'NONE',  #18472 ) ;
#10239=EDGE_CURVE ( 'NONE', #15949, #8848, #11333, .T. ) ;
#10240=DIRECTION ( 'NONE',  ( 1.000000000000000000, 0.000000000000000000, -1.124692329640370702E-16 ) ) ;
#10264=LINE ( 'NONE', #3390, #9315 ) ;
#10285=VERTEX_POINT ( 'NONE', #8133 ) ;
#10309=ADVANCED_FACE ( 'NONE', ( #19581 ), #8448, .T. ) ;
#10313=VERTEX_POINT ( 'NONE', #18012 ) ;
#10318=EDGE_CURVE ( 'NONE', #11249, #3359, #300, .T. ) ;
#10339=ORIENTED_EDGE ( 'NONE', *, *, #15388, .F. ) ;
#10359=ORIENTED_EDGE ( 'NONE', *, *, #10239, .F. ) ;
#10389=FACE_OUTER_BOUND ( 'NONE', #11806, .T. ) ;
#10407=ADVANCED_FACE ( 'NONE', ( #8875 ), #2527, .F. ) ;
#10451=CARTESIAN_POINT ( 'NONE',  ( 32.39721438298033007, 261.8427481158985302, -5.999999999999973355 ) ) ;
#10454=DIRECTION ( 'NONE',  ( -0.8660254037844370423, -0.5000000000000027756, -1.818545872641207967E-15 ) ) ;
#10523=ADVANCED_FACE ( 'NONE', ( #4629, #20626, #11096 ), #17569, .T. ) ;
#10552=ORIENTED_EDGE ( 'NONE', *, *, #7559, .T. ) ;
#10556=DIRECTION ( 'NONE',  ( 0.5000000000000041078, -0.8660254037844363761, 0.000000000000000000 ) ) ;
#10579=ORIENTED_EDGE ( 'NONE', *, *, #20804, .F. ) ;
#10606=DIRECTION ( 'NONE',  ( 0.5000000000000029976, -0.8660254037844370423, 0.000000000000000000 ) ) ;
#10615=LINE ( 'NONE', #20471, #8114 ) ;
#10629=LINE ( 'NONE', #5959, #1750 ) ;
#10642=LINE ( 'NONE', #17126, #3705 ) ;
#10648=ORIENTED_EDGE ( 'NONE', *, *, #7773, .F. ) ;
#10650=CARTESIAN_POINT ( 'NONE',  ( 44.21948262095328630, 217.3659788670219370, 44.53282986889900030 ) ) ;
#10671=DIRECTION ( 'NONE',  ( -0.3841106397986888688, 0.6652991438591145945, -0.6401843996644803747 ) ) ;
#10683=VECTOR ( 'NONE', #5616, 1000.000000000000000 ) ;
#10721=DIRECTION ( 'NONE',  ( -0.8660254037844360431, -0.5000000000000044409, 5.976026924694052093E-17 ) ) ;
#10730=LINE ( 'NONE', #17210, #19688 ) ;
#10769=FACE_OUTER_BOUND ( 'NONE', #2670, .T. ) ;
#10776=EDGE_CURVE ( 'NONE', #3810, #15949, #11266, .T. ) ;
#10807=ORIENTED_EDGE ( 'NONE', *, *, #15838, .F. ) ;
#10810=VERTEX_POINT ( 'NONE', #10650 ) ;
#10834=LINE ( 'NONE', #9033, #6756 ) ;
#10862=CARTESIAN_POINT ( 'NONE',  ( 34.99529059433363898, 263.3427481158985302, -22.00000000000000355 ) ) ;
#10913=DIRECTION ( 'NONE',  ( 0.000000000000000000, -0.8108848540793835991, 0.5852057359806522863 ) ) ;
#11034=VERTEX_POINT ( 'NONE', #18276 ) ;
#11057=EDGE_CURVE ( 'NONE', #10810, #19247, #16477, .T. ) ;
#11077=DIRECTION ( 'NONE',  ( -0.8660254037844360431, -0.5000000000000044409, 5.976026924694052093E-17 ) ) ;
#11090=VERTEX_POINT ( 'NONE', #5428 ) ;
#11091=CIRCLE ( 'NONE', #17193, 5.000000000000002665 ) ;
#11096=FACE_BOUND ( 'NONE', #17794, .T. ) ;
#11110=ORIENTED_EDGE ( 'NONE', *, *, #11057, .F. ) ;
#11134=CIRCLE ( 'NONE', #17909, 5.000000000000001776 ) ;
#11146=AXIS2_PLACEMENT_3D ( 'NONE', #19896, #5470, #17910 ) ;
#11217=ORIENTED_EDGE ( 'NONE', *, *, #17858, .F. ) ;
#11219=CARTESIAN_POINT ( 'NONE',  ( 48.48114019555096377, 209.9845714233581191, 45.12705109663953351 ) ) ;
#11249=VERTEX_POINT ( 'NONE', #4065 ) ;
#11254=CARTESIAN_POINT ( 'NONE',  ( 89.99529059433416478, 168.0799536996104848, 21.00000000000000711 ) ) ;
#11257=LINE ( 'NONE', #943, #18905 ) ;
#11262=CARTESIAN_POINT ( 'NONE',  ( 82.49529059433407951, 181.0703347563770365, 11.00000000000001066 ) ) ;
#11266=CIRCLE ( 'NONE', #18039, 5.000000000000005329 ) ;
#11287=ORIENTED_EDGE ( 'NONE', *, *, #17549, .T. ) ;
#11289=LINE ( 'NONE', #4400, #18962 ) ;
#11291=VERTEX_POINT ( 'NONE', #3286 ) ;
#11333=LINE ( 'NONE', #6745, #10190 ) ;
#11346=ORIENTED_EDGE ( 'NONE', *, *, #17858, .T. ) ;
#11354=DIRECTION ( 'NONE',  ( -0.8660254037844360431, -0.5000000000000044409, 0.000000000000000000 ) ) ;
#11484=EDGE_CURVE ( 'NONE', #15901, #1882, #18002, .T. ) ;
#11502=PLANE ( 'NONE',  #5546 ) ;
#11537=DIRECTION ( 'NONE',  ( 1.051300182579813185E-16, -6.256999452958517077E-17, 1.000000000000000000 ) ) ;
#11540=VECTOR ( 'NONE', #20745, 1000.000000000000227 ) ;
#11547=VERTEX_POINT ( 'NONE', #11219 ) ;
#11584=EDGE_LOOP ( 'NONE', ( #524, #6074, #4818, #10579 ) ) ;
#11594=EDGE_CURVE ( 'NONE', #3757, #3717, #4605, .T. ) ;
#11618=EDGE_CURVE ( 'NONE', #8848, #15901, #14058, .T. ) ;
#11620=EDGE_CURVE ( 'NONE', #13841, #16063, #4188, .T. ) ;
#11635=CARTESIAN_POINT ( 'NONE',  ( 83.78935635788883474, 148.8289471055651063, 58.21056266367804000 ) ) ;
#11649=CARTESIAN_POINT ( 'NONE',  ( 99.99529059433426426, 150.7594456239217777, 21.00000000000000711 ) ) ;
#11651=CARTESIAN_POINT ( 'NONE',  ( 22.32500173739932237, 255.2883321626825932, 8.042028396309266469 ) ) ;
#11681=ORIENTED_EDGE ( 'NONE', *, *, #3494, .T. ) ;
#11705=CARTESIAN_POINT ( 'NONE',  ( 35.31538279416582071, 262.7883321626826501, 8.042028396309232718 ) ) ;
#11744=CARTESIAN_POINT ( 'NONE',  ( 42.39721438298049350, 244.5222400402098231, -18.99999999999997513 ) ) ;
#11746=DIRECTION ( 'NONE',  ( -1.129794457510891260E-16, 7.616560175797575475E-17, -1.000000000000000000 ) ) ;
#11749=EDGE_CURVE ( 'NONE', #6648, #3810, #14483, .T. ) ;
#11757=DIRECTION ( 'NONE',  ( 0.5000000000000046629, -0.8660254037844360431, 0.000000000000000000 ) ) ;
#11765=ORIENTED_EDGE ( 'NONE', *, *, #3270, .T. ) ;
#11774=CARTESIAN_POINT ( 'NONE',  ( 137.6791466197848592, 79.48909236273166812, 1.792808077408215874E-16 ) ) ;
#11806=EDGE_LOOP ( 'NONE', ( #19021, #18762, #20181, #953 ) ) ;
#11874=ORIENTED_EDGE ( 'NONE', *, *, #2292, .T. ) ;
#11876=AXIS2_PLACEMENT_3D ( 'NONE', #15477, #16735, #5794 ) ;
#11906=CYLINDRICAL_SURFACE ( 'NONE', #19560, 5.000000000000002665 ) ;
#11930=AXIS2_PLACEMENT_3D ( 'NONE', #3370, #11537, #5161 ) ;
#11934=( NAMED_UNIT ( * ) PLANE_ANGLE_UNIT ( ) SI_UNIT ( $, .RADIAN. ) );
#11956=CARTESIAN_POINT ( 'NONE',  ( 69.50490953756755630, 173.5703347563769796, 16.00000000000001066 ) ) ;
#11972=DIRECTION ( 'NONE',  ( -0.3841106397986904786, 0.6652991438591134843, -0.6401843996644803747 ) ) ;
#11991=ADVANCED_FACE ( 'NONE', ( #466 ), #16682, .F. ) ;
#11995=ORIENTED_EDGE ( 'NONE', *, *, #10239, .T. ) ;
#12016=DIRECTION ( 'NONE',  ( -0.8660254037844361541, -0.5000000000000045519, 5.976026924694054558E-17 ) ) ;
#12033=EDGE_CURVE ( 'NONE', #17073, #8802, #20266, .T. ) ;
#12048=ORIENTED_EDGE ( 'NONE', *, *, #14090, .F. ) ;
#12054=PLANE ( 'NONE',  #17319 ) ;
#12070=CARTESIAN_POINT ( 'NONE',  ( -83.06735915341819521, 143.8768865042907521, 44.53282986889873740 ) ) ;
#12112=DIRECTION ( 'NONE',  ( -0.8660254037844360431, -0.5000000000000044409, 5.976026924694052093E-17 ) ) ;
#12152=CARTESIAN_POINT ( 'NONE',  ( 164.5049095375683521, 9.025508037334198264, -14.00000000000000355 ) ) ;
#12169=DIRECTION ( 'NONE',  ( 5.175391130484829193E-17, 2.988013462347053780E-17, 1.000000000000000000 ) ) ;
#12187=ORIENTED_EDGE ( 'NONE', *, *, #2019, .F. ) ;
#12198=CARTESIAN_POINT ( 'NONE',  ( 34.99529059433363898, 263.3427481158985302, -5.999999999999973355 ) ) ;
#12219=( LENGTH_UNIT ( ) NAMED_UNIT ( * ) SI_UNIT ( .MILLI., .METRE. ) );
#12237=DIRECTION ( 'NONE',  ( 0.5000000000000058842, -0.8660254037844352659, 0.000000000000000000 ) ) ;
#12283=VECTOR ( 'NONE', #988, 1000.000000000000114 ) ;
#12330=PLANE ( 'NONE',  #7234 ) ;
#12348=CARTESIAN_POINT ( 'NONE',  ( 172.3972143829816162, 19.35563505625646030, -14.00000000000000533 ) ) ;
#12355=PRODUCT_DEFINITION_CONTEXT ( 'detailed design', #2851, 'design' ) ;
#12374=ORIENTED_EDGE ( 'NONE', *, *, #14090, .T. ) ;
#12402=ORIENTED_EDGE ( 'NONE', *, *, #7150, .T. ) ;
#12408=ORIENTED_EDGE ( 'NONE', *, *, #11057, .T. ) ;
#12442=CARTESIAN_POINT ( 'NONE',  ( 34.99529059433364608, 263.3427481158985302, 1.000000000000017097 ) ) ;
#12487=CARTESIAN_POINT ( 'NONE',  ( 87.00490953756771262, 143.2594456239216925, 21.00000000000000711 ) ) ;
#12526=ORIENTED_EDGE ( 'NONE', *, *, #2414, .T. ) ;
#12549=DIRECTION ( 'NONE',  ( 0.000000000000000000, 0.000000000000000000, -1.000000000000000000 ) ) ;
#12554=DIRECTION ( 'NONE',  ( -1.000000000000000000, 0.000000000000000000, 1.218100516808353647E-16 ) ) ;
#12561=LINE ( 'NONE', #7664, #10198 ) ;
#12618=LINE ( 'NONE', #16282, #6554 ) ;
#12643=ORIENTED_EDGE ( 'NONE', *, *, #3186, .F. ) ;
#12655=ORIENTED_EDGE ( 'NONE', *, *, #1732, .T. ) ;
#12711=CARTESIAN_POINT ( 'NONE',  ( 82.49529059433407951, 181.0703347563770365, 16.00000000000001066 ) ) ;
#12796=VECTOR ( 'NONE', #9974, 1000.000000000000227 ) ;
#12837=EDGE_LOOP ( 'NONE', ( #3218, #10648, #2043, #4326 ) ) ;
#12846=LINE ( 'NONE', #14664, #6539 ) ;
#12896=VECTOR ( 'NONE', #10721, 1000.000000000000227 ) ;
#12960=PLANE ( 'NONE',  #13578 ) ;
#12975=ORIENTED_EDGE ( 'NONE', *, *, #20804, .T. ) ;
#12982=DIRECTION ( 'NONE',  ( -0.8660254037844361541, -0.5000000000000045519, 5.976026924694053325E-17 ) ) ;
#13059=FACE_OUTER_BOUND ( 'NONE', #15393, .T. ) ;
#13081=ORIENTED_EDGE ( 'NONE', *, *, #9977, .T. ) ;
#13097=EDGE_LOOP ( 'NONE', ( #6341, #4378, #14209, #11874, #4693, #16408, #8499, #1792 ) ) ;
#13103=PLANE ( 'NONE',  #20172 ) ;
#13106=FACE_OUTER_BOUND ( 'NONE', #1938, .T. ) ;
#13135=VECTOR ( 'NONE', #1451, 1000.000000000000227 ) ;
#13181=CARTESIAN_POINT ( 'NONE',  ( 172.3972143829816162, 19.35563505625646030, -14.00000000000000533 ) ) ;
#13191=DIRECTION ( 'NONE',  ( -0.5000000000000042188, 0.8660254037844361541, 1.401122807519728636E-16 ) ) ;
#13197=EDGE_CURVE ( 'NONE', #1744, #16111, #17989, .T. ) ;
#13202=ORIENTED_EDGE ( 'NONE', *, *, #16480, .F. ) ;
#13249=CARTESIAN_POINT ( 'NONE',  ( 87.00490953756771262, 143.2594456239216925, 21.00000000000000711 ) ) ;
#13271=PLANE ( 'NONE',  #15726 ) ;
#13276=PLANE ( 'NONE',  #8473 ) ;
#13280=ORIENTED_EDGE ( 'NONE', *, *, #17202, .F. ) ;
#13282=EDGE_CURVE ( 'NONE', #5897, #2748, #596, .T. ) ;
#13360=ORIENTED_EDGE ( 'NONE', *, *, #16276, .T. ) ;
#13375=LINE ( 'NONE', #6572, #715 ) ;
#13407=AXIS2_PLACEMENT_3D ( 'NONE', #15391, #8987, #4015 ) ;
#13446=LINE ( 'NONE', #16831, #20217 ) ;
#13459=ORIENTED_EDGE ( 'NONE', *, *, #12033, .F. ) ;
#13495=DIRECTION ( 'NONE',  ( 0.000000000000000000, 0.000000000000000000, 1.000000000000000000 ) ) ;
#13517=LINE ( 'NONE', #19963, #2775 ) ;
#13544=VERTEX_POINT ( 'NONE', #3609 ) ;
#13553=DIRECTION ( 'NONE',  ( -0.8660254037844360431, -0.5000000000000044409, 5.976026924694052093E-17 ) ) ;
#13578=AXIS2_PLACEMENT_3D ( 'NONE', #7953, #17730, #11354 ) ;
#13610=ORIENTED_EDGE ( 'NONE', *, *, #17317, .F. ) ;
#13676=CARTESIAN_POINT ( 'NONE',  ( 89.99529059433416478, 168.0799536996104848, 26.00000000000001066 ) ) ;
#13678=ADVANCED_FACE ( 'NONE', ( #7212 ), #13271, .F. ) ;
#13734=ORIENTED_EDGE ( 'NONE', *, *, #814, .T. ) ;
#13754=CARTESIAN_POINT ( 'NONE',  ( 172.0049095375684090, -3.964873019432338275, -29.00000000000001066 ) ) ;
#13799=ORIENTED_EDGE ( 'NONE', *, *, #10164, .F. ) ;
#13815=LINE ( 'NONE', #12442, #12896 ) ;
#13841=VERTEX_POINT ( 'NONE', #6439 ) ;
#13845=ORIENTED_EDGE ( 'NONE', *, *, #11484, .F. ) ;
#13855=CARTESIAN_POINT ( 'NONE',  ( 89.99529059433416478, 168.0799536996104848, 26.00000000000001066 ) ) ;
#13880=VERTEX_POINT ( 'NONE', #14334 ) ;
#13907=DIRECTION ( 'NONE',  ( -0.8660254037844361541, -0.5000000000000045519, 5.976026924694053325E-17 ) ) ;
#13909=VECTOR ( 'NONE', #14876, 1000.000000000000114 ) ;
#13932=CARTESIAN_POINT ( 'NONE',  ( 42.39721438298049350, 244.5222400402098231, -8.999999999999973355 ) ) ;
#13954=ORIENTED_EDGE ( 'NONE', *, *, #5736, .F. ) ;
#13975=CARTESIAN_POINT ( 'NONE',  ( 77.00490953756764156, 160.5799536996104280, 21.00000000000000711 ) ) ;
#13979=ORIENTED_EDGE ( 'NONE', *, *, #1148, .T. ) ;
#14058=LINE ( 'NONE', #15655, #7510 ) ;
#14063=EDGE_CURVE ( 'NONE', #16111, #3757, #19180, .T. ) ;
#14090=EDGE_CURVE ( 'NONE', #19247, #11249, #15171, .T. ) ;
#14094=ORIENTED_EDGE ( 'NONE', *, *, #14998, .T. ) ;
#14107=ORIENTED_EDGE ( 'NONE', *, *, #17317, .T. ) ;
#14208=EDGE_LOOP ( 'NONE', ( #92, #17986, #8983, #2489, #13799, #16917, #2838, #5901, #7217, #3365, #10807, #17089 ) ) ;
#14209=ORIENTED_EDGE ( 'NONE', *, *, #873, .F. ) ;
#14236=ORIENTED_EDGE ( 'NONE', *, *, #2843, .T. ) ;
#14238=ORIENTED_EDGE ( 'NONE', *, *, #2837, .T. ) ;
#14334=CARTESIAN_POINT ( 'NONE',  ( 184.9952905943349606, 3.535126980567709687, -6.000000000000009770 ) ) ;
#14386=CARTESIAN_POINT ( 'NONE',  ( 99.99529059433426426, 150.7594456239217777, 1.000000000000006883 ) ) ;
#14387=DIRECTION ( 'NONE',  ( -0.5000000000000057732, 0.8660254037844353769, 0.000000000000000000 ) ) ;
#14390=EDGE_LOOP ( 'NONE', ( #14473, #19295, #19231, #10 ) ) ;
#14393=VERTEX_POINT ( 'NONE', #5446 ) ;
#14404=DIRECTION ( 'NONE',  ( -0.8660254037844360431, -0.5000000000000044409, 5.976026924694052093E-17 ) ) ;
#14408=ORIENTED_EDGE ( 'NONE', *, *, #19516, .F. ) ;
#14441=CIRCLE ( 'NONE', #8990, 5.000000000000001776 ) ;
#14442=ORIENTED_EDGE ( 'NONE', *, *, #3270, .F. ) ;
#14473=ORIENTED_EDGE ( 'NONE', *, *, #13197, .T. ) ;
#14483=LINE ( 'NONE', #19336, #6827 ) ;
#14485=DIRECTION ( 'NONE',  ( -0.8660254037844360431, -0.5000000000000044409, 5.976026924694052093E-17 ) ) ;
#14499=VECTOR ( 'NONE', #13553, 1000.000000000000227 ) ;
#14547=EDGE_LOOP ( 'NONE', ( #14107, #2768, #2432, #4475 ) ) ;
#14549=DIRECTION ( 'NONE',  ( -0.3200921998322431850, 0.5544159532159285142, 0.7682212795973754060 ) ) ;
#14558=CARTESIAN_POINT ( 'NONE',  ( 162.0049095375683237, 13.35563505625637859, -14.00000000000000355 ) ) ;
#14565=ORIENTED_EDGE ( 'NONE', *, *, #16152, .F. ) ;
#14653=ORIENTED_EDGE ( 'NONE', *, *, #15838, .T. ) ;
#14661=AXIS2_PLACEMENT_3D ( 'NONE', #12487, #20425, #3039 ) ;
#14664=CARTESIAN_POINT ( 'NONE',  ( 34.99529059433364608, 263.3427481158985302, -28.99999999999997513 ) ) ;
#14714=ORIENTED_EDGE ( 'NONE', *, *, #19505, .T. ) ;
#14732=EDGE_LOOP ( 'NONE', ( #14653, #9710, #9913, #7081 ) ) ;
#14744=FACE_OUTER_BOUND ( 'NONE', #20866, .T. ) ;
#14750=LINE ( 'NONE', #3681, #362 ) ;
#14767=DIRECTION ( 'NONE',  ( 0.5000000000000043299, -0.8660254037844361541, 0.000000000000000000 ) ) ;
#14818=EDGE_CURVE ( 'NONE', #5234, #1744, #7540, .T. ) ;
#14876=DIRECTION ( 'NONE',  ( -0.8660254037844370423, -0.5000000000000027756, -1.818545872641207967E-15 ) ) ;
#14881=DIRECTION ( 'NONE',  ( -0.8660254037844360431, -0.5000000000000044409, 5.976026924694052093E-17 ) ) ;
#14882=EDGE_CURVE ( 'NONE', #16846, #16240, #17592, .T. ) ;
#14890=CARTESIAN_POINT ( 'NONE',  ( 34.99529059433364608, 263.3427481158985302, -28.99999999999997513 ) ) ;
#14949=DIRECTION ( 'NONE',  ( 0.5000000000000044409, -0.8660254037844360431, 0.000000000000000000 ) ) ;
#14998=EDGE_CURVE ( 'NONE', #16413, #13880, #10264, .T. ) ;
#14999=LINE ( 'NONE', #352, #9341 ) ;
#15057=LINE ( 'NONE', #7067, #14499 ) ;
#15111=VECTOR ( 'NONE', #19307, 1000.000000000000114 ) ;
#15162=LINE ( 'NONE', #8557, #16485 ) ;
#15171=LINE ( 'NONE', #18118, #5611 ) ;
#15186=PRODUCT_DEFINITION_SHAPE ( 'NONE', 'NONE',  #7172 ) ;
#15205=ADVANCED_FACE ( 'NONE', ( #8915 ), #18362, .F. ) ;
#15217=CARTESIAN_POINT ( 'NONE',  ( 82.49529059433407951, 181.0703347563770365, 6.000000000000009770 ) ) ;
#15235=CARTESIAN_POINT ( 'NONE',  ( 184.9952905943349606, 3.535126980567713240, 0.9999999999999876765 ) ) ;
#15255=EDGE_CURVE ( 'NONE', #16063, #13880, #7219, .T. ) ;
#15274=FACE_OUTER_BOUND ( 'NONE', #10138, .T. ) ;
#15348=ORIENTED_EDGE ( 'NONE', *, *, #5613, .T. ) ;
#15385=VECTOR ( 'NONE', #1871, 1000.000000000000000 ) ;
#15388=EDGE_CURVE ( 'NONE', #5897, #10313, #14441, .T. ) ;
#15391=CARTESIAN_POINT ( 'NONE',  ( 44.99529059433372424, 246.0222400402097946, -13.99999999999997513 ) ) ;
#15393=EDGE_LOOP ( 'NONE', ( #5016, #13954, #17656, #209 ) ) ;
#15395=ADVANCED_FACE ( 'NONE', ( #3381 ), #16222, .T. ) ;
#15465=LINE ( 'NONE', #13754, #19668 ) ;
#15477=CARTESIAN_POINT ( 'NONE',  ( 52.00490953756739287, 203.8812238888322383, 11.00000000000001066 ) ) ;
#15502=DIRECTION ( 'NONE',  ( -0.5000000000000045519, 0.8660254037844360431, 0.000000000000000000 ) ) ;
#15522=( NAMED_UNIT ( * ) SI_UNIT ( $, .STERADIAN. ) SOLID_ANGLE_UNIT ( ) );
#15527=ADVANCED_FACE ( 'NONE', ( #7193 ), #740, .F. ) ;
#15541=VERTEX_POINT ( 'NONE', #5487 ) ;
#15550=CARTESIAN_POINT ( 'NONE',  ( 46.88067919638974956, 212.7566511894377754, 48.96815749462641065 ) ) ;
#15630=CARTESIAN_POINT ( 'NONE',  ( 182.3972143829816446, 2.035126980567696364, -22.00000000000003908 ) ) ;
#15655=CARTESIAN_POINT ( 'NONE',  ( 174.9952905943348469, 20.85563505625644609, -19.00000000000000355 ) ) ;
#15679=CARTESIAN_POINT ( 'NONE',  ( 32.39721438298033007, 261.8427481158985302, -22.00000000000000355 ) ) ;
#15711=DIRECTION ( 'NONE',  ( 0.000000000000000000, 0.000000000000000000, 1.000000000000000000 ) ) ;
#15726=AXIS2_PLACEMENT_3D ( 'NONE', #2141, #544, #19928 ) ;
#15796=DIRECTION ( 'NONE',  ( -1.000000000000000000, 0.000000000000000000, 5.175391130484829193E-17 ) ) ;
#15828=DIRECTION ( 'NONE',  ( -0.8660254037844360431, -0.5000000000000044409, 5.976026924694052093E-17 ) ) ;
#15838=EDGE_CURVE ( 'NONE', #1208, #1744, #18005, .T. ) ;
#15860=DIRECTION ( 'NONE',  ( -0.5000000000000043299, 0.8660254037844361541, 1.272130549049658454E-16 ) ) ;
#15891=ORIENTED_EDGE ( 'NONE', *, *, #15255, .F. ) ;
#15900=CIRCLE ( 'NONE', #8071, 5.000000000000005329 ) ;
#15901=VERTEX_POINT ( 'NONE', #817 ) ;
#15903=CARTESIAN_POINT ( 'NONE',  ( 0.000000000000000000, 0.000000000000000000, 0.000000000000000000 ) ) ;
#15934=DIRECTION ( 'NONE',  ( -0.5000000000000057732, 0.8660254037844353769, 0.000000000000000000 ) ) ;
#15936=CARTESIAN_POINT ( 'NONE',  ( 99.99529059433426426, 150.7594456239217777, 21.00000000000000711 ) ) ;
#15949=VERTEX_POINT ( 'NONE', #11744 ) ;
#16036=SHAPE_DEFINITION_REPRESENTATION ( #15186, #20473 ) ;
#16045=FACE_OUTER_BOUND ( 'NONE', #614, .T. ) ;
#16063=VERTEX_POINT ( 'NONE', #4205 ) ;
#16069=CARTESIAN_POINT ( 'NONE',  ( 34.99529059433363898, 263.3427481158985302, -5.999999999999973355 ) ) ;
#16072=LINE ( 'NONE', #14386, #3417 ) ;
#16105=EDGE_LOOP ( 'NONE', ( #16631, #3412, #7546, #6731 ) ) ;
#16108=DIRECTION ( 'NONE',  ( 0.8660254037844360431, 0.5000000000000044409, -5.976026924694053325E-17 ) ) ;
#16111=VERTEX_POINT ( 'NONE', #13975 ) ;
#16143=CARTESIAN_POINT ( 'NONE',  ( 48.48114019555096377, 209.9845714233581191, 45.12705109663953351 ) ) ;
#16152=EDGE_CURVE ( 'NONE', #16560, #7294, #17140, .T. ) ;
#16154=DIRECTION ( 'NONE',  ( -0.000000000000000000, -0.000000000000000000, -1.000000000000000000 ) ) ;
#16164=ORIENTED_EDGE ( 'NONE', *, *, #17990, .F. ) ;
#16222=PLANE ( 'NONE',  #877 ) ;
#16240=VERTEX_POINT ( 'NONE', #19441 ) ;
#16276=EDGE_CURVE ( 'NONE', #1882, #16846, #8352, .T. ) ;
#16282=CARTESIAN_POINT ( 'NONE',  ( 82.49529059433407951, 181.0703347563770365, 16.00000000000001066 ) ) ;
#16361=UNCERTAINTY_MEASURE_WITH_UNIT (LENGTH_MEASURE( 1.000000000000000082E-05 ), #12219, 'distance_accuracy_value', 'NONE');
#16362=EDGE_LOOP ( 'NONE', ( #4191, #12402, #11287, #14714 ) ) ;
#16408=ORIENTED_EDGE ( 'NONE', *, *, #2260, .F. ) ;
#16413=VERTEX_POINT ( 'NONE', #19964 ) ;
#16457=VECTOR ( 'NONE', #3473, 1000.000000000000114 ) ;
#16477=LINE ( 'NONE', #1960, #7493 ) ;
#16480=EDGE_CURVE ( 'NONE', #10313, #11034, #8000, .T. ) ;
#16485=VECTOR ( 'NONE', #18314, 1000.000000000000227 ) ;
#16498=VERTEX_POINT ( 'NONE', #11254 ) ;
#16560=VERTEX_POINT ( 'NONE', #1808 ) ;
#16566=DIRECTION ( 'NONE',  ( 0.5000000000000057732, -0.8660254037844353769, 0.000000000000000000 ) ) ;
#16594=ORIENTED_EDGE ( 'NONE', *, *, #6008, .T. ) ;
#16620=AXIS2_PLACEMENT_3D ( 'NONE', #12711, #4439, #15796 ) ;
#16622=CIRCLE ( 'NONE', #3405, 5.000000000000002665 ) ;
#16631=ORIENTED_EDGE ( 'NONE', *, *, #7593, .F. ) ;
#16682=PLANE ( 'NONE',  #9872 ) ;
#16702=( LENGTH_UNIT ( ) NAMED_UNIT ( * ) SI_UNIT ( .MILLI., .METRE. ) );
#16703=DIRECTION ( 'NONE',  ( -0.8660254037844360431, -0.5000000000000044409, 5.976026924694052093E-17 ) ) ;
#16709=DIRECTION ( 'NONE',  ( 0.8660254037844361541, 0.5000000000000043299, 3.166650901095681677E-16 ) ) ;
#16735=DIRECTION ( 'NONE',  ( 0.8660254037844360431, 0.5000000000000044409, -5.976026924694053325E-17 ) ) ;
#16775=CLOSED_SHELL ( 'NONE', ( #19580, #17658, #11991, #19003, #10523, #1012, #443, #17387, #9333, #19606, #102, #2386, #15527, #18076, #17612, #10309, #18987, #19131, #15205, #5503, #13678, #10407, #18532, #1496, #8866, #15395, #6819, #7699 ) ) ;
#16781=VECTOR ( 'NONE', #12112, 1000.000000000000227 ) ;
#16831=CARTESIAN_POINT ( 'NONE',  ( 49.99529059433375267, 237.3619860023654553, 26.00000000000001776 ) ) ;
#16846=VERTEX_POINT ( 'NONE', #4239 ) ;
#16847=ORIENTED_EDGE ( 'NONE', *, *, #2260, .T. ) ;
#16856=VECTOR ( 'NONE', #8073, 1000.000000000000114 ) ;
#16896=ORIENTED_EDGE ( 'NONE', *, *, #1582, .F. ) ;
#16910=AXIS2_PLACEMENT_3D ( 'NONE', #5678, #12169, #18633 ) ;
#16917=ORIENTED_EDGE ( 'NONE', *, *, #9866, .F. ) ;
#17017=EDGE_LOOP ( 'NONE', ( #5229, #19764, #11765, #8353 ) ) ;
#17073=VERTEX_POINT ( 'NONE', #10124 ) ;
#17086=VECTOR ( 'NONE', #18429, 1000.000000000000000 ) ;
#17089=ORIENTED_EDGE ( 'NONE', *, *, #19516, .T. ) ;
#17126=CARTESIAN_POINT ( 'NONE',  ( 34.99529059433364608, 263.3427481158985302, -28.99999999999997513 ) ) ;
#17140=LINE ( 'NONE', #5883, #5957 ) ;
#17144=EDGE_CURVE ( 'NONE', #10285, #5234, #13446, .T. ) ;
#17176=LINE ( 'NONE', #20553, #5456 ) ;
#17193=AXIS2_PLACEMENT_3D ( 'NONE', #19339, #8079, #14387 ) ;
#17197=EDGE_CURVE ( 'NONE', #11090, #11291, #15162, .T. ) ;
#17202=EDGE_CURVE ( 'NONE', #5086, #8157, #15057, .T. ) ;
#17210=CARTESIAN_POINT ( 'NONE',  ( 22.00490953756710510, 255.8427481158984733, -28.99999999999997513 ) ) ;
#17242=DIRECTION ( 'NONE',  ( 0.8660254037844361541, 0.5000000000000043299, -5.976026924694053325E-17 ) ) ;
#17252=VECTOR ( 'NONE', #5454, 1000.000000000000227 ) ;
#17294=CARTESIAN_POINT ( 'NONE',  ( 174.8972143829816446, 15.02550803733428353, -14.00000000000000533 ) ) ;
#17306=CIRCLE ( 'NONE', #10178, 5.000000000000001776 ) ;
#17317=EDGE_CURVE ( 'NONE', #17073, #16560, #3034, .T. ) ;
#17319=AXIS2_PLACEMENT_3D ( 'NONE', #13855, #20303, #18728 ) ;
#17327=AXIS2_PLACEMENT_3D ( 'NONE', #8200, #3232, #1650 ) ;
#17345=EDGE_LOOP ( 'NONE', ( #10339, #16896, #6370, #17817, #13202 ) ) ;
#17387=ADVANCED_FACE ( 'NONE', ( #4828 ), #19354, .F. ) ;
#17458=ORIENTED_EDGE ( 'NONE', *, *, #3186, .T. ) ;
#17489=DIRECTION ( 'NONE',  ( 0.5000000000000043299, -0.8660254037844361541, -1.401122807519728883E-16 ) ) ;
#17549=EDGE_CURVE ( 'NONE', #122, #11547, #5750, .T. ) ;
#17562=DIRECTION ( 'NONE',  ( 0.5000000000000045519, -0.8660254037844361541, 0.000000000000000000 ) ) ;
#17569=PLANE ( 'NONE',  #14661 ) ;
#17592=LINE ( 'NONE', #6328, #20239 ) ;
#17612=ADVANCED_FACE ( 'NONE', ( #4804 ), #42, .F. ) ;
#17636=ORIENTED_EDGE ( 'NONE', *, *, #13282, .F. ) ;
#17656=ORIENTED_EDGE ( 'NONE', *, *, #9514, .F. ) ;
#17658=ADVANCED_FACE ( 'NONE', ( #10389 ), #11906, .F. ) ;
#17730=DIRECTION ( 'NONE',  ( -0.5000000000000045519, 0.8660254037844361541, 4.006172263299079574E-16 ) ) ;
#17741=MANIFOLD_SOLID_BREP ( 'Chamfer3', #16775 ) ;
#17794=EDGE_LOOP ( 'NONE', ( #2854, #2312, #15348, #13081, #2217 ) ) ;
#17817=ORIENTED_EDGE ( 'NONE', *, *, #5912, .F. ) ;
#17827=DIRECTION ( 'NONE',  ( 0.8660254037844360431, 0.5000000000000044409, -5.976026924694053325E-17 ) ) ;
#17855=DIRECTION ( 'NONE',  ( 0.5000000000000057732, -0.8660254037844353769, 0.000000000000000000 ) ) ;
#17857=LINE ( 'NONE', #16069, #20792 ) ;
#17858=EDGE_CURVE ( 'NONE', #19247, #14393, #11257, .T. ) ;
#17885=ORIENTED_EDGE ( 'NONE', *, *, #8711, .T. ) ;
#17909=AXIS2_PLACEMENT_3D ( 'NONE', #12348, #18801, #12237 ) ;
#17910=DIRECTION ( 'NONE',  ( 0.5000000000000029976, -0.8660254037844370423, 0.000000000000000000 ) ) ;
#17980=CARTESIAN_POINT ( 'NONE',  ( -43.39423452328062325, 75.16101894988052834, 104.1461628558723760 ) ) ;
#17982=VERTEX_POINT ( 'NONE', #7440 ) ;
#17986=ORIENTED_EDGE ( 'NONE', *, *, #9145, .T. ) ;
#17989=LINE ( 'NONE', #9904, #15385 ) ;
#17990=EDGE_CURVE ( 'NONE', #8848, #5086, #11134, .T. ) ;
#18002=LINE ( 'NONE', #3470, #3441 ) ;
#18005=LINE ( 'NONE', #6528, #16457 ) ;
#18012=CARTESIAN_POINT ( 'NONE',  ( 84.99529059433410794, 176.7402077374548526, 11.00000000000001066 ) ) ;
#18039=AXIS2_PLACEMENT_3D ( 'NONE', #8657, #8551, #10556 ) ;
#18076=ADVANCED_FACE ( 'NONE', ( #3113 ), #7659, .T. ) ;
#18113=DIRECTION ( 'NONE',  ( -0.8660254037844361541, -0.5000000000000042188, -3.026831728535680894E-16 ) ) ;
#18118=CARTESIAN_POINT ( 'NONE',  ( 33.39482959517242477, 266.1148278819781581, 4.841106397986906451 ) ) ;
#18167=CARTESIAN_POINT ( 'NONE',  ( 172.0049095375684090, -3.964873019432352486, 0.9999999999999885647 ) ) ;
#18170=AXIS2_PLACEMENT_3D ( 'NONE', #3440, #20923, #4720 ) ;
#18191=CARTESIAN_POINT ( 'NONE',  ( 172.3972143829816162, 19.35563505625646741, -9.000000000000007105 ) ) ;
#18226=CARTESIAN_POINT ( 'NONE',  ( -44.99469552244184456, 77.93309871596017047, 107.9872692538592531 ) ) ;
#18233=AXIS2_PLACEMENT_3D ( 'NONE', #15903, #1274, #19656 ) ;
#18276=CARTESIAN_POINT ( 'NONE',  ( 82.49529059433407951, 181.0703347563770365, 6.000000000000009770 ) ) ;
#18277=CARTESIAN_POINT ( 'NONE',  ( 184.9952905943349606, 3.535126980567727450, -29.00000000000001066 ) ) ;
#18314=DIRECTION ( 'NONE',  ( -0.8660254037844360431, -0.5000000000000044409, 5.976026924694052093E-17 ) ) ;
#18337=CIRCLE ( 'NONE', #17327, 5.000000000000001776 ) ;
#18346=FACE_BOUND ( 'NONE', #5551, .T. ) ;
#18359=CARTESIAN_POINT ( 'NONE',  ( 64.99529059433395162, 211.3812238888322952, 16.00000000000001066 ) ) ;
#18362=CYLINDRICAL_SURFACE ( 'NONE', #3559, 5.000000000000001776 ) ;
#18377=DIRECTION ( 'NONE',  ( 0.5000000000000044409, -0.8660254037844360431, 0.000000000000000000 ) ) ;
#18429=DIRECTION ( 'NONE',  ( 0.000000000000000000, 0.000000000000000000, 1.000000000000000000 ) ) ;
#18436=ORIENTED_EDGE ( 'NONE', *, *, #1148, .F. ) ;
#18463=CARTESIAN_POINT ( 'NONE',  ( 64.99529059433392320, 211.3812238888322952, 11.00000000000001066 ) ) ;
#18466=EDGE_CURVE ( 'NONE', #11090, #4169, #15900, .T. ) ;
#18468=DIRECTION ( 'NONE',  ( -0.8660254037844360431, -0.5000000000000043299, 0.000000000000000000 ) ) ;
#18472=AXIS2_PLACEMENT_3D ( 'NONE', #2205, #11746, #7066 ) ;
#18480=DIRECTION ( 'NONE',  ( -0.5000000000000045519, 0.8660254037844360431, 0.000000000000000000 ) ) ;
#18525=FACE_OUTER_BOUND ( 'NONE', #19803, .T. ) ;
#18532=ADVANCED_FACE ( 'NONE', ( #18346, #222 ), #6985, .F. ) ;
#18539=EDGE_LOOP ( 'NONE', ( #10359, #12975, #13845, #3415 ) ) ;
#18579=FACE_OUTER_BOUND ( 'NONE', #8330, .T. ) ;
#18584=CARTESIAN_POINT ( 'NONE',  ( 59.87106025315629410, 220.2566511894378039, 48.96815749462643197 ) ) ;
#18602=ORIENTED_EDGE ( 'NONE', *, *, #11618, .T. ) ;
#18633=DIRECTION ( 'NONE',  ( 1.000000000000000000, 0.000000000000000000, -5.175391130484829193E-17 ) ) ;
#18643=FACE_OUTER_BOUND ( 'NONE', #16362, .T. ) ;
#18661=CIRCLE ( 'NONE', #3758, 19.99999999999999645 ) ;
#18714=CARTESIAN_POINT ( 'NONE',  ( 32.00490953756718682, 238.5222400402097662, -18.99999999999997513 ) ) ;
#18728=DIRECTION ( 'NONE',  ( -0.8660254037844360431, -0.5000000000000044409, 0.000000000000000000 ) ) ;
#18762=ORIENTED_EDGE ( 'NONE', *, *, #17202, .T. ) ;
#18801=DIRECTION ( 'NONE',  ( -0.8660254037844360431, -0.5000000000000043299, 0.000000000000000000 ) ) ;
#18843=PLANE ( 'NONE',  #16910 ) ;
#18894=DIRECTION ( 'NONE',  ( 1.153604387573318063E-16, -8.028960261725416899E-17, 1.000000000000000000 ) ) ;
#18905=VECTOR ( 'NONE', #7386, 1000.000000000000114 ) ;
#18962=VECTOR ( 'NONE', #11077, 1000.000000000000227 ) ;
#18987=ADVANCED_FACE ( 'NONE', ( #517 ), #6962, .F. ) ;
#19003=ADVANCED_FACE ( 'NONE', ( #14744, #8344 ), #198, .F. ) ;
#19021=ORIENTED_EDGE ( 'NONE', *, *, #814, .F. ) ;
#19123=ORIENTED_EDGE ( 'NONE', *, *, #873, .T. ) ;
#19131=ADVANCED_FACE ( 'NONE', ( #10769 ), #18843, .T. ) ;
#19160=CARTESIAN_POINT ( 'NONE',  ( 64.99529059433392320, 211.3812238888322952, 16.00000000000001066 ) ) ;
#19170=ORIENTED_EDGE ( 'NONE', *, *, #4592, .F. ) ;
#19180=CIRCLE ( 'NONE', #1912, 19.99999999999999645 ) ;
#19198=PRODUCT_CONTEXT ( 'NONE', #123, 'mechanical' ) ;
#19205=ADVANCED_BREP_SHAPE_REPRESENTATION ( '', ( #17741, #18233 ), #20925 ) ;
#19210=LINE ( 'NONE', #5082, #1218 ) ;
#19231=ORIENTED_EDGE ( 'NONE', *, *, #8711, .F. ) ;
#19239=ORIENTED_EDGE ( 'NONE', *, *, #9145, .F. ) ;
#19247=VERTEX_POINT ( 'NONE', #5991 ) ;
#19295=ORIENTED_EDGE ( 'NONE', *, *, #20399, .F. ) ;
#19299=CARTESIAN_POINT ( 'NONE',  ( 82.49529059433407951, 181.0703347563770365, 11.00000000000001066 ) ) ;
#19307=DIRECTION ( 'NONE',  ( 0.8660254037844370423, 0.5000000000000027756, 1.850371707708595943E-15 ) ) ;
#19336=CARTESIAN_POINT ( 'NONE',  ( 42.39721438298049350, 244.5222400402098231, -8.999999999999973355 ) ) ;
#19339=CARTESIAN_POINT ( 'NONE',  ( 162.0049095375683237, 13.35563505625637859, -14.00000000000000355 ) ) ;
#19354=PLANE ( 'NONE',  #7018 ) ;
#19387=CARTESIAN_POINT ( 'NONE',  ( 72.00490953756758472, 169.2402077374547957, 11.00000000000001243 ) ) ;
#19423=EDGE_LOOP ( 'NONE', ( #5797, #20168, #1527, #3735 ) ) ;
#19441=CARTESIAN_POINT ( 'NONE',  ( 162.0049095375683237, 13.35563505625637859, -9.000000000000005329 ) ) ;
#19503=CYLINDRICAL_SURFACE ( 'NONE', #3914, 19.99999999999999645 ) ;
#19505=EDGE_CURVE ( 'NONE', #11547, #17982, #6665, .T. ) ;
#19516=EDGE_CURVE ( 'NONE', #1208, #11547, #19210, .T. ) ;
#19545=DIRECTION ( 'NONE',  ( 0.8660254037844360431, 0.5000000000000044409, 0.000000000000000000 ) ) ;
#19547=DIRECTION ( 'NONE',  ( -1.000000000000000000, 0.000000000000000000, 9.512199820426880209E-17 ) ) ;
#19560=AXIS2_PLACEMENT_3D ( 'NONE', #19735, #7117, #16566 ) ;
#19563=ORIENTED_EDGE ( 'NONE', *, *, #8198, .T. ) ;
#19571=LINE ( 'NONE', #9814, #6447 ) ;
#19574=ORIENTED_EDGE ( 'NONE', *, *, #4592, .T. ) ;
#19580=ADVANCED_FACE ( 'NONE', ( #16045 ), #9848, .F. ) ;
#19581=FACE_OUTER_BOUND ( 'NONE', #18539, .T. ) ;
#19599=ORIENTED_EDGE ( 'NONE', *, *, #11620, .T. ) ;
#19606=ADVANCED_FACE ( 'NONE', ( #13059 ), #19503, .F. ) ;
#19626=VECTOR ( 'NONE', #14404, 1000.000000000000227 ) ;
#19656=DIRECTION ( 'NONE',  ( 1.000000000000000000, 0.000000000000000000, 0.000000000000000000 ) ) ;
#19668=VECTOR ( 'NONE', #5673, 1000.000000000000000 ) ;
#19688=VECTOR ( 'NONE', #9036, 1000.000000000000227 ) ;
#19735=CARTESIAN_POINT ( 'NONE',  ( 174.9952905943348469, 20.85563505625644609, -14.00000000000000533 ) ) ;
#19764=ORIENTED_EDGE ( 'NONE', *, *, #16480, .T. ) ;
#19778=VERTEX_POINT ( 'NONE', #540 ) ;
#19798=DIRECTION ( 'NONE',  ( -0.8660254037844360431, -0.5000000000000044409, 5.976026924694053325E-17 ) ) ;
#19803=EDGE_LOOP ( 'NONE', ( #7737, #2358, #9506, #1554 ) ) ;
#19831=VERTEX_POINT ( 'NONE', #12198 ) ;
#19896=CARTESIAN_POINT ( 'NONE',  ( 82.49529059433407951, 181.0703347563770365, 11.00000000000001066 ) ) ;
#19928=DIRECTION ( 'NONE',  ( -1.000000000000000000, 0.000000000000000000, 1.153604387573317816E-16 ) ) ;
#19963=CARTESIAN_POINT ( 'NONE',  ( 34.99529059433364608, 263.3427481158985302, 1.000000000000028644 ) ) ;
#19964=CARTESIAN_POINT ( 'NONE',  ( 182.3972143829816730, 2.035126980567732780, -5.999999999999974243 ) ) ;
#20075=ORIENTED_EDGE ( 'NONE', *, *, #14998, .F. ) ;
#20099=VERTEX_POINT ( 'NONE', #909 ) ;
#20109=ORIENTED_EDGE ( 'NONE', *, *, #14882, .T. ) ;
#20140=CARTESIAN_POINT ( 'NONE',  ( 34.99529059433364608, 263.3427481158985302, -28.99999999999997513 ) ) ;
#20152=CARTESIAN_POINT ( 'NONE',  ( 184.9952905943349606, 3.535126980567727450, -29.00000000000001066 ) ) ;
#20159=CARTESIAN_POINT ( 'NONE',  ( 89.99529059433416478, 168.0799536996104848, 26.00000000000001066 ) ) ;
#20168=ORIENTED_EDGE ( 'NONE', *, *, #3595, .T. ) ;
#20172=AXIS2_PLACEMENT_3D ( 'NONE', #1757, #17562, #19545 ) ;
#20181=ORIENTED_EDGE ( 'NONE', *, *, #2414, .F. ) ;
#20194=PLANE ( 'NONE',  #4770 ) ;
#20217=VECTOR ( 'NONE', #721, 1000.000000000000114 ) ;
#20237=PRODUCT ( 'Drill Bit Assembly Sliding Track Base', 'Drill Bit Assembly Sliding Track Base', '', ( #19198 ) ) ;
#20239=VECTOR ( 'NONE', #17489, 1000.000000000000114 ) ;
#20248=EDGE_CURVE ( 'NONE', #8157, #15901, #11091, .T. ) ;
#20266=LINE ( 'NONE', #15630, #6161 ) ;
#20303=DIRECTION ( 'NONE',  ( -0.5000000000000045519, 0.8660254037844361541, 0.000000000000000000 ) ) ;
#20323=DIRECTION ( 'NONE',  ( -0.08515265670862154357, 0.1474887278187986539, 0.9853913436913560586 ) ) ;
#20345=VECTOR ( 'NONE', #3776, 1000.000000000000000 ) ;
#20366=DIRECTION ( 'NONE',  ( 1.000000000000000000, 0.000000000000000000, -1.153604387573318063E-16 ) ) ;
#20399=EDGE_CURVE ( 'NONE', #16498, #16111, #1848, .T. ) ;
#20425=DIRECTION ( 'NONE',  ( -0.8660254037844361541, -0.5000000000000045519, 5.976026924694054558E-17 ) ) ;
#20431=ORIENTED_EDGE ( 'NONE', *, *, #12033, .T. ) ;
#20448=CARTESIAN_POINT ( 'NONE',  ( 44.99529059433372424, 246.0222400402097946, -18.99999999999997513 ) ) ;
#20471=CARTESIAN_POINT ( 'NONE',  ( 34.99529059433364608, 263.3427481158985302, -28.99999999999997513 ) ) ;
#20473=SHAPE_REPRESENTATION ( 'Drill Bit Assembly Sliding Track Base', ( #18233 ), #20925 ) ;
#20539=PLANE ( 'NONE',  #16620 ) ;
#20553=CARTESIAN_POINT ( 'NONE',  ( 22.00490953756710510, 255.8427481158984733, -28.99999999999997513 ) ) ;
#20606=ORIENTED_EDGE ( 'NONE', *, *, #2292, .F. ) ;
#20609=DIRECTION ( 'NONE',  ( 0.000000000000000000, 0.000000000000000000, 1.000000000000000000 ) ) ;
#20626=FACE_BOUND ( 'NONE', #9630, .T. ) ;
#20660=VECTOR ( 'NONE', #15860, 1000.000000000000227 ) ;
#20716=CARTESIAN_POINT ( 'NONE',  ( 99.99529059433426426, 150.7594456239217777, 1.000000000000008438 ) ) ;
#20745=DIRECTION ( 'NONE',  ( -0.8660254037844360431, -0.5000000000000044409, 5.976026924694052093E-17 ) ) ;
#20792=VECTOR ( 'NONE', #7981, 1000.000000000000227 ) ;
#20804=EDGE_CURVE ( 'NONE', #15949, #1882, #5700, .T. ) ;
#20866=EDGE_LOOP ( 'NONE', ( #12048, #11346, #16594, #17458, #5220, #17885, #7160, #19599, #2631, #12187, #11681, #8429 ) ) ;
#20923=DIRECTION ( 'NONE',  ( 0.8660254037844360431, 0.5000000000000044409, -5.976026924694053325E-17 ) ) ;
#20925=( GEOMETRIC_REPRESENTATION_CONTEXT ( 3 ) GLOBAL_UNCERTAINTY_ASSIGNED_CONTEXT ( ( #243 ) ) GLOBAL_UNIT_ASSIGNED_CONTEXT ( ( #16702, #11934, #3645 ) ) REPRESENTATION_CONTEXT ( 'NONE', 'WORKASPACE' ) );
#20961=COLOUR_RGB('Dark Blue',0.08,0.2,0.34);
#20962=FILL_AREA_STYLE_COLOUR('',#20961);
#20963=FILL_AREA_STYLE('',(#20962));
#20964=SURFACE_STYLE_FILL_AREA(#20963);
#20965=SURFACE_SIDE_STYLE('',(#20964));
#20966=SURFACE_STYLE_USAGE(.BOTH.,#20965);
#20967=PRESENTATION_STYLE_ASSIGNMENT((#20966));
ENDSEC;
END-ISO-10303-21;
